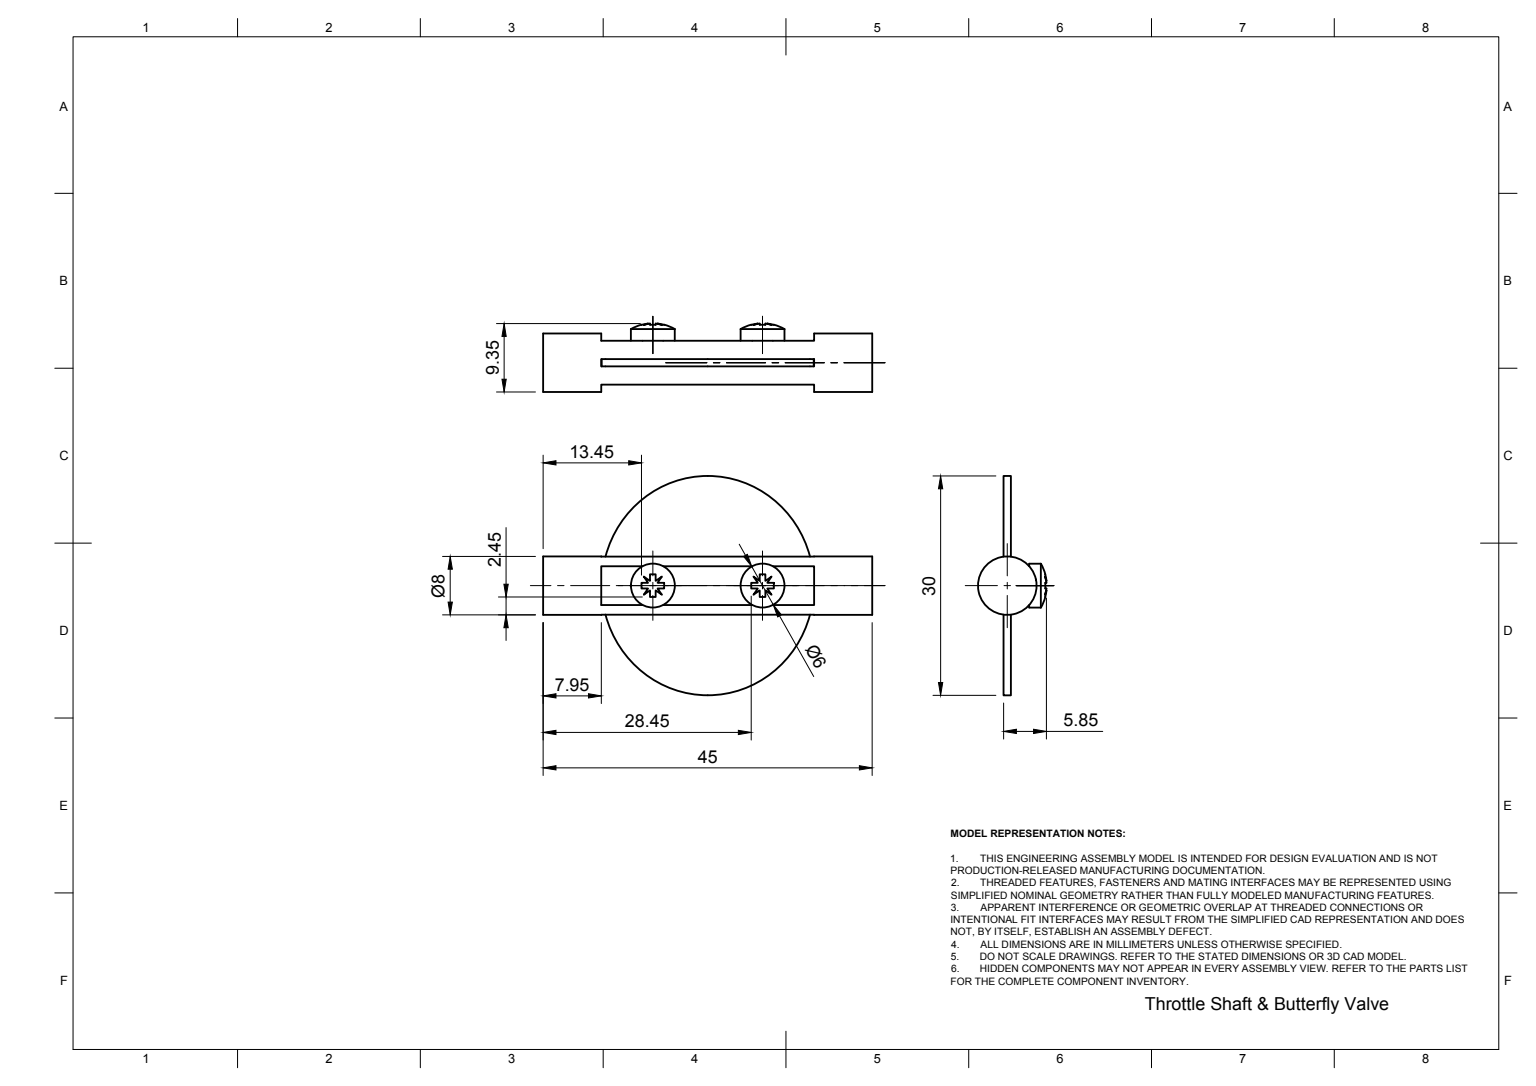
ISO-10303-21;
HEADER;
/* Generated by software containing ST-Developer
 * from STEP Tools, Inc. (www.steptools.com) 
 */

FILE_DESCRIPTION(
/* description */ ('STEP AP214'),
/* implementation_level */ '2;1');

FILE_NAME(
/* name */ 'Throttle Shaft & Butterfly Valve.step',
/* time_stamp */ '2026-10-07T12:18:07-07:00',
/* author */ (''),
/* organization */ (''),
/* preprocessor_version */ 'ST-DEVELOPER v20.2',
/* originating_system */ 'Autodesk Translation Framework v15.15.0.0',
/* authorisation */ '');

FILE_SCHEMA (('AUTOMOTIVE_DESIGN { 1 0 10303 214 3 1 1 }'));
ENDSEC;

DATA;
#10=MECHANICAL_DESIGN_GEOMETRIC_PRESENTATION_REPRESENTATION('',(#124),#62974);
#80=SPHERICAL_SURFACE('',#15545,6.);
#81=SPHERICAL_SURFACE('',#15579,6.);
#100=SHAPE_REPRESENTATION_RELATIONSHIP('SRR','None',#63023,#112);
#112=ADVANCED_BREP_SHAPE_REPRESENTATION('',(#136),#62964);
#124=STYLED_ITEM('',(#63090),#136);
#136=MANIFOLD_SOLID_BREP('Body1',#15194);
#147=(
BOUNDED_SURFACE()
B_SPLINE_SURFACE(3,1,((#34070,#34071),(#34072,#34073),(#34074,#34075),(#34076,
#34077)),.UNSPECIFIED.,.F.,.F.,.F.)
B_SPLINE_SURFACE_WITH_KNOTS((4,4),(2,2),(0.,1.),(0.,0.12),.UNSPECIFIED.)
GEOMETRIC_REPRESENTATION_ITEM()
RATIONAL_B_SPLINE_SURFACE(((1.,1.),(0.333333333333333,0.333333333333333),
(0.333333333333333,0.333333333333333),(1.,1.)))
REPRESENTATION_ITEM('')
SURFACE()
);
#148=(
BOUNDED_SURFACE()
B_SPLINE_SURFACE(3,1,((#34465,#34466),(#34467,#34468),(#34469,#34470),(#34471,
#34472)),.UNSPECIFIED.,.F.,.F.,.F.)
B_SPLINE_SURFACE_WITH_KNOTS((4,4),(2,2),(0.,1.),(0.,0.120000000000004),
 .UNSPECIFIED.)
GEOMETRIC_REPRESENTATION_ITEM()
RATIONAL_B_SPLINE_SURFACE(((1.,1.),(0.333333333333333,0.333333333333333),
(0.333333333333333,0.333333333333333),(1.,1.)))
REPRESENTATION_ITEM('')
SURFACE()
);
#212=FACE_BOUND('',#4694,.T.);
#213=FACE_BOUND('',#4696,.T.);
#214=FACE_BOUND('',#4697,.T.);
#215=FACE_BOUND('',#4698,.T.);
#216=FACE_BOUND('',#4700,.T.);
#365=PLANE('',#15607);
#366=PLANE('',#15609);
#367=PLANE('',#15610);
#368=PLANE('',#15612);
#369=PLANE('',#15613);
#370=PLANE('',#15614);
#371=PLANE('',#15615);
#372=PLANE('',#15616);
#373=PLANE('',#15617);
#374=PLANE('',#15618);
#375=PLANE('',#15619);
#376=PLANE('',#15620);
#377=PLANE('',#15621);
#378=PLANE('',#15622);
#379=PLANE('',#15623);
#380=PLANE('',#15624);
#381=PLANE('',#15625);
#382=PLANE('',#15626);
#383=PLANE('',#15627);
#384=PLANE('',#15628);
#385=PLANE('',#15629);
#386=PLANE('',#15630);
#387=PLANE('',#15631);
#388=PLANE('',#15632);
#389=PLANE('',#15633);
#390=PLANE('',#15634);
#391=PLANE('',#15635);
#392=PLANE('',#15636);
#393=PLANE('',#15637);
#394=PLANE('',#15638);
#395=PLANE('',#15639);
#396=PLANE('',#15640);
#397=PLANE('',#15641);
#398=PLANE('',#15642);
#399=PLANE('',#15643);
#400=PLANE('',#15644);
#401=PLANE('',#15645);
#402=PLANE('',#15646);
#403=PLANE('',#15647);
#404=PLANE('',#15648);
#405=PLANE('',#15649);
#406=PLANE('',#15650);
#407=PLANE('',#15651);
#408=PLANE('',#15652);
#409=PLANE('',#15653);
#410=PLANE('',#15654);
#411=PLANE('',#15655);
#412=PLANE('',#15656);
#413=PLANE('',#15657);
#414=PLANE('',#15658);
#415=PLANE('',#15659);
#416=PLANE('',#15660);
#417=PLANE('',#15661);
#418=PLANE('',#15662);
#419=PLANE('',#15663);
#420=PLANE('',#15664);
#421=PLANE('',#15665);
#422=PLANE('',#15666);
#423=PLANE('',#15667);
#424=PLANE('',#15668);
#425=PLANE('',#15669);
#426=PLANE('',#15670);
#427=PLANE('',#15671);
#428=PLANE('',#15673);
#429=PLANE('',#15675);
#430=PLANE('',#15678);
#739=ELLIPSE('',#15532,14.9999999999992,14.4999999999993);
#740=ELLIPSE('',#15533,15.0000000000004,14.5000000000004);
#741=ELLIPSE('',#15534,14.9999999999913,14.4999999999828);
#742=ELLIPSE('',#15535,15.0000000000001,14.5000000000001);
#743=ELLIPSE('',#15536,15.,14.5);
#744=ELLIPSE('',#15537,14.9999999999864,14.4999999999732);
#745=ELLIPSE('',#15608,14.9999999999937,14.4999999999875);
#746=ELLIPSE('',#15611,15.0000000000065,14.5000000000128);
#747=ELLIPSE('',#15672,15.0000000000007,14.5000000000006);
#748=ELLIPSE('',#15674,15.0000000000004,14.5000000000003);
#749=ELLIPSE('',#15676,15.0000000000002,14.5000000000001);
#750=ELLIPSE('',#15677,15.0000000000002,14.5000000000002);
#1237=LINE('',#34082,#2430);
#1238=LINE('',#34090,#2431);
#1239=LINE('',#34103,#2432);
#1240=LINE('',#34153,#2433);
#1241=LINE('',#34156,#2434);
#1242=LINE('',#34158,#2435);
#1243=LINE('',#34160,#2436);
#1244=LINE('',#34164,#2437);
#1245=LINE('',#34169,#2438);
#1246=LINE('',#34170,#2439);
#1247=LINE('',#34172,#2440);
#1248=LINE('',#34178,#2441);
#1249=LINE('',#34179,#2442);
#1250=LINE('',#34181,#2443);
#1251=LINE('',#34184,#2444);
#1252=LINE('',#34186,#2445);
#1253=LINE('',#34187,#2446);
#1254=LINE('',#34192,#2447);
#1255=LINE('',#34195,#2448);
#1256=LINE('',#34199,#2449);
#1257=LINE('',#34200,#2450);
#1258=LINE('',#34202,#2451);
#1259=LINE('',#34204,#2452);
#1260=LINE('',#34206,#2453);
#1261=LINE('',#34210,#2454);
#1262=LINE('',#34212,#2455);
#1263=LINE('',#34213,#2456);
#1264=LINE('',#34214,#2457);
#1265=LINE('',#34215,#2458);
#1266=LINE('',#34264,#2459);
#1267=LINE('',#34269,#2460);
#1268=LINE('',#34271,#2461);
#1269=LINE('',#34274,#2462);
#1270=LINE('',#34278,#2463);
#1271=LINE('',#34280,#2464);
#1272=LINE('',#34281,#2465);
#1273=LINE('',#34284,#2466);
#1274=LINE('',#34285,#2467);
#1275=LINE('',#34288,#2468);
#1276=LINE('',#34290,#2469);
#1277=LINE('',#34292,#2470);
#1278=LINE('',#34294,#2471);
#1279=LINE('',#34296,#2472);
#1280=LINE('',#34298,#2473);
#1281=LINE('',#34300,#2474);
#1282=LINE('',#34302,#2475);
#1283=LINE('',#34304,#2476);
#1284=LINE('',#34306,#2477);
#1285=LINE('',#34308,#2478);
#1286=LINE('',#34310,#2479);
#1287=LINE('',#34312,#2480);
#1288=LINE('',#34314,#2481);
#1289=LINE('',#34316,#2482);
#1290=LINE('',#34318,#2483);
#1291=LINE('',#34320,#2484);
#1292=LINE('',#34321,#2485);
#1293=LINE('',#34323,#2486);
#1294=LINE('',#34324,#2487);
#1295=LINE('',#34326,#2488);
#1296=LINE('',#34328,#2489);
#1297=LINE('',#34330,#2490);
#1298=LINE('',#34332,#2491);
#1299=LINE('',#34334,#2492);
#1300=LINE('',#34336,#2493);
#1301=LINE('',#34338,#2494);
#1302=LINE('',#34340,#2495);
#1303=LINE('',#34342,#2496);
#1304=LINE('',#34344,#2497);
#1305=LINE('',#34346,#2498);
#1306=LINE('',#34348,#2499);
#1307=LINE('',#34350,#2500);
#1308=LINE('',#34352,#2501);
#1309=LINE('',#34354,#2502);
#1310=LINE('',#34359,#2503);
#1311=LINE('',#34363,#2504);
#1312=LINE('',#34367,#2505);
#1313=LINE('',#34371,#2506);
#1314=LINE('',#34373,#2507);
#1315=LINE('',#34379,#2508);
#1316=LINE('',#34381,#2509);
#1317=LINE('',#34383,#2510);
#1318=LINE('',#34385,#2511);
#1319=LINE('',#34387,#2512);
#1320=LINE('',#34389,#2513);
#1321=LINE('',#34391,#2514);
#1322=LINE('',#34393,#2515);
#1323=LINE('',#34395,#2516);
#1324=LINE('',#34397,#2517);
#1325=LINE('',#34399,#2518);
#1326=LINE('',#34401,#2519);
#1327=LINE('',#34403,#2520);
#1328=LINE('',#34405,#2521);
#1329=LINE('',#34407,#2522);
#1330=LINE('',#34409,#2523);
#1331=LINE('',#34411,#2524);
#1332=LINE('',#34413,#2525);
#1333=LINE('',#34415,#2526);
#1334=LINE('',#34416,#2527);
#1335=LINE('',#34418,#2528);
#1336=LINE('',#34419,#2529);
#1337=LINE('',#34421,#2530);
#1338=LINE('',#34423,#2531);
#1339=LINE('',#34425,#2532);
#1340=LINE('',#34427,#2533);
#1341=LINE('',#34429,#2534);
#1342=LINE('',#34431,#2535);
#1343=LINE('',#34433,#2536);
#1344=LINE('',#34435,#2537);
#1345=LINE('',#34437,#2538);
#1346=LINE('',#34439,#2539);
#1347=LINE('',#34441,#2540);
#1348=LINE('',#34443,#2541);
#1349=LINE('',#34445,#2542);
#1350=LINE('',#34447,#2543);
#1351=LINE('',#34449,#2544);
#1352=LINE('',#34451,#2545);
#1353=LINE('',#34453,#2546);
#1354=LINE('',#34455,#2547);
#2430=VECTOR('',#17528,1000.);
#2431=VECTOR('',#17535,1000.);
#2432=VECTOR('',#17548,3.);
#2433=VECTOR('',#17601,4.);
#2434=VECTOR('',#17604,1000.);
#2435=VECTOR('',#17605,1000.);
#2436=VECTOR('',#17606,1000.);
#2437=VECTOR('',#17609,4.);
#2438=VECTOR('',#17614,1000.);
#2439=VECTOR('',#17615,1000.);
#2440=VECTOR('',#17616,1000.);
#2441=VECTOR('',#17621,1000.);
#2442=VECTOR('',#17622,1000.);
#2443=VECTOR('',#17623,1000.);
#2444=VECTOR('',#17626,1000.);
#2445=VECTOR('',#17627,1000.);
#2446=VECTOR('',#17628,1000.);
#2447=VECTOR('',#17631,1000.);
#2448=VECTOR('',#17634,1000.);
#2449=VECTOR('',#17637,1000.);
#2450=VECTOR('',#17638,1000.);
#2451=VECTOR('',#17639,1000.);
#2452=VECTOR('',#17640,1000.);
#2453=VECTOR('',#17641,1000.);
#2454=VECTOR('',#17644,1000.);
#2455=VECTOR('',#17645,1000.);
#2456=VECTOR('',#17646,1000.);
#2457=VECTOR('',#17647,1000.);
#2458=VECTOR('',#17648,1000.);
#2459=VECTOR('',#17701,3.);
#2460=VECTOR('',#17710,1000.);
#2461=VECTOR('',#17713,1000.);
#2462=VECTOR('',#17718,1000.);
#2463=VECTOR('',#17723,1000.);
#2464=VECTOR('',#17724,1000.);
#2465=VECTOR('',#17725,1000.);
#2466=VECTOR('',#17728,1000.);
#2467=VECTOR('',#17729,1000.);
#2468=VECTOR('',#17732,1000.);
#2469=VECTOR('',#17733,1000.);
#2470=VECTOR('',#17734,1000.);
#2471=VECTOR('',#17735,1000.);
#2472=VECTOR('',#17736,1000.);
#2473=VECTOR('',#17737,1000.);
#2474=VECTOR('',#17738,1000.);
#2475=VECTOR('',#17739,1000.);
#2476=VECTOR('',#17740,1000.);
#2477=VECTOR('',#17741,1000.);
#2478=VECTOR('',#17742,1000.);
#2479=VECTOR('',#17743,1000.);
#2480=VECTOR('',#17744,1000.);
#2481=VECTOR('',#17745,1000.);
#2482=VECTOR('',#17746,1000.);
#2483=VECTOR('',#17747,1000.);
#2484=VECTOR('',#17748,1000.);
#2485=VECTOR('',#17749,1000.);
#2486=VECTOR('',#17752,1000.);
#2487=VECTOR('',#17753,1000.);
#2488=VECTOR('',#17756,1000.);
#2489=VECTOR('',#17759,1000.);
#2490=VECTOR('',#17762,1000.);
#2491=VECTOR('',#17765,1000.);
#2492=VECTOR('',#17768,1000.);
#2493=VECTOR('',#17771,1000.);
#2494=VECTOR('',#17774,1000.);
#2495=VECTOR('',#17777,1000.);
#2496=VECTOR('',#17780,1000.);
#2497=VECTOR('',#17783,1000.);
#2498=VECTOR('',#17786,1000.);
#2499=VECTOR('',#17789,1000.);
#2500=VECTOR('',#17792,1000.);
#2501=VECTOR('',#17795,1000.);
#2502=VECTOR('',#17798,1000.);
#2503=VECTOR('',#17807,1000.);
#2504=VECTOR('',#17814,1000.);
#2505=VECTOR('',#17821,1000.);
#2506=VECTOR('',#17828,1000.);
#2507=VECTOR('',#17831,1000.);
#2508=VECTOR('',#17838,1000.);
#2509=VECTOR('',#17839,1000.);
#2510=VECTOR('',#17840,1000.);
#2511=VECTOR('',#17841,1000.);
#2512=VECTOR('',#17842,1000.);
#2513=VECTOR('',#17843,1000.);
#2514=VECTOR('',#17844,1000.);
#2515=VECTOR('',#17845,1000.);
#2516=VECTOR('',#17846,1000.);
#2517=VECTOR('',#17847,1000.);
#2518=VECTOR('',#17848,1000.);
#2519=VECTOR('',#17849,1000.);
#2520=VECTOR('',#17850,1000.);
#2521=VECTOR('',#17851,1000.);
#2522=VECTOR('',#17852,1000.);
#2523=VECTOR('',#17853,1000.);
#2524=VECTOR('',#17854,1000.);
#2525=VECTOR('',#17855,1000.);
#2526=VECTOR('',#17856,1000.);
#2527=VECTOR('',#17857,1000.);
#2528=VECTOR('',#17860,1000.);
#2529=VECTOR('',#17861,1000.);
#2530=VECTOR('',#17864,1000.);
#2531=VECTOR('',#17867,1000.);
#2532=VECTOR('',#17870,1000.);
#2533=VECTOR('',#17873,1000.);
#2534=VECTOR('',#17876,1000.);
#2535=VECTOR('',#17879,1000.);
#2536=VECTOR('',#17882,1000.);
#2537=VECTOR('',#17885,1000.);
#2538=VECTOR('',#17888,1000.);
#2539=VECTOR('',#17891,1000.);
#2540=VECTOR('',#17894,1000.);
#2541=VECTOR('',#17897,1000.);
#2542=VECTOR('',#17900,1000.);
#2543=VECTOR('',#17903,1000.);
#2544=VECTOR('',#17906,1000.);
#2545=VECTOR('',#17909,1000.);
#2546=VECTOR('',#17912,1000.);
#2547=VECTOR('',#17915,1000.);
#3461=CYLINDRICAL_SURFACE('',#15538,3.);
#3462=CYLINDRICAL_SURFACE('',#15566,4.);
#3463=CYLINDRICAL_SURFACE('',#15601,3.);
#3806=FACE_OUTER_BOUND('',#4691,.T.);
#3807=FACE_OUTER_BOUND('',#4692,.T.);
#3808=FACE_OUTER_BOUND('',#4693,.T.);
#3809=FACE_OUTER_BOUND('',#4695,.T.);
#3810=FACE_OUTER_BOUND('',#4699,.T.);
#3811=FACE_OUTER_BOUND('',#4701,.T.);
#3812=FACE_OUTER_BOUND('',#4702,.T.);
#3813=FACE_OUTER_BOUND('',#4703,.T.);
#3814=FACE_OUTER_BOUND('',#4704,.T.);
#3815=FACE_OUTER_BOUND('',#4705,.T.);
#3816=FACE_OUTER_BOUND('',#4706,.T.);
#3817=FACE_OUTER_BOUND('',#4707,.T.);
#3818=FACE_OUTER_BOUND('',#4708,.T.);
#3819=FACE_OUTER_BOUND('',#4709,.T.);
#3820=FACE_OUTER_BOUND('',#4710,.T.);
#3821=FACE_OUTER_BOUND('',#4711,.T.);
#3822=FACE_OUTER_BOUND('',#4712,.T.);
#3823=FACE_OUTER_BOUND('',#4713,.T.);
#3824=FACE_OUTER_BOUND('',#4714,.T.);
#3825=FACE_OUTER_BOUND('',#4715,.T.);
#3826=FACE_OUTER_BOUND('',#4716,.T.);
#3827=FACE_OUTER_BOUND('',#4717,.T.);
#3828=FACE_OUTER_BOUND('',#4718,.T.);
#3829=FACE_OUTER_BOUND('',#4719,.T.);
#3830=FACE_OUTER_BOUND('',#4720,.T.);
#3831=FACE_OUTER_BOUND('',#4721,.T.);
#3832=FACE_OUTER_BOUND('',#4722,.T.);
#3833=FACE_OUTER_BOUND('',#4723,.T.);
#3834=FACE_OUTER_BOUND('',#4724,.T.);
#3835=FACE_OUTER_BOUND('',#4725,.T.);
#3836=FACE_OUTER_BOUND('',#4726,.T.);
#3837=FACE_OUTER_BOUND('',#4727,.T.);
#3838=FACE_OUTER_BOUND('',#4728,.T.);
#3839=FACE_OUTER_BOUND('',#4729,.T.);
#3840=FACE_OUTER_BOUND('',#4730,.T.);
#3841=FACE_OUTER_BOUND('',#4731,.T.);
#3842=FACE_OUTER_BOUND('',#4732,.T.);
#3843=FACE_OUTER_BOUND('',#4733,.T.);
#3844=FACE_OUTER_BOUND('',#4734,.T.);
#3845=FACE_OUTER_BOUND('',#4735,.T.);
#3846=FACE_OUTER_BOUND('',#4736,.T.);
#3847=FACE_OUTER_BOUND('',#4737,.T.);
#3848=FACE_OUTER_BOUND('',#4738,.T.);
#3849=FACE_OUTER_BOUND('',#4739,.T.);
#3850=FACE_OUTER_BOUND('',#4740,.T.);
#3851=FACE_OUTER_BOUND('',#4741,.T.);
#3852=FACE_OUTER_BOUND('',#4742,.T.);
#3853=FACE_OUTER_BOUND('',#4743,.T.);
#3854=FACE_OUTER_BOUND('',#4744,.T.);
#3855=FACE_OUTER_BOUND('',#4745,.T.);
#3856=FACE_OUTER_BOUND('',#4746,.T.);
#3857=FACE_OUTER_BOUND('',#4747,.T.);
#3858=FACE_OUTER_BOUND('',#4748,.T.);
#3859=FACE_OUTER_BOUND('',#4749,.T.);
#3860=FACE_OUTER_BOUND('',#4750,.T.);
#3861=FACE_OUTER_BOUND('',#4751,.T.);
#3862=FACE_OUTER_BOUND('',#4752,.T.);
#3863=FACE_OUTER_BOUND('',#4753,.T.);
#3864=FACE_OUTER_BOUND('',#4754,.T.);
#3865=FACE_OUTER_BOUND('',#4755,.T.);
#3866=FACE_OUTER_BOUND('',#4756,.T.);
#3867=FACE_OUTER_BOUND('',#4757,.T.);
#3868=FACE_OUTER_BOUND('',#4758,.T.);
#3869=FACE_OUTER_BOUND('',#4759,.T.);
#3870=FACE_OUTER_BOUND('',#4760,.T.);
#3871=FACE_OUTER_BOUND('',#4761,.T.);
#3872=FACE_OUTER_BOUND('',#4762,.T.);
#3873=FACE_OUTER_BOUND('',#4763,.T.);
#3874=FACE_OUTER_BOUND('',#4764,.T.);
#3875=FACE_OUTER_BOUND('',#4765,.T.);
#3876=FACE_OUTER_BOUND('',#4766,.T.);
#3877=FACE_OUTER_BOUND('',#4767,.T.);
#3878=FACE_OUTER_BOUND('',#4768,.T.);
#4691=EDGE_LOOP('',(#10355,#10356,#10357,#10358,#10359,#10360,#10361,#10362));
#4692=EDGE_LOOP('',(#10363,#10364,#10365,#10366,#10367,#10368,#10369,#10370));
#4693=EDGE_LOOP('',(#10371));
#4694=EDGE_LOOP('',(#10372,#10373,#10374,#10375,#10376,#10377,#10378,#10379,
#10380,#10381,#10382,#10383,#10384,#10385,#10386,#10387,#10388,#10389,#10390,
#10391));
#4695=EDGE_LOOP('',(#10392,#10393,#10394,#10395,#10396,#10397,#10398,#10399,
#10400,#10401,#10402,#10403,#10404,#10405,#10406,#10407));
#4696=EDGE_LOOP('',(#10408,#10409,#10410,#10411,#10412,#10413,#10414,#10415));
#4697=EDGE_LOOP('',(#10416,#10417,#10418,#10419));
#4698=EDGE_LOOP('',(#10420,#10421,#10422,#10423,#10424,#10425,#10426,#10427,
#10428,#10429,#10430,#10431));
#4699=EDGE_LOOP('',(#10432));
#4700=EDGE_LOOP('',(#10433,#10434,#10435,#10436,#10437,#10438,#10439,#10440,
#10441,#10442,#10443,#10444,#10445,#10446,#10447,#10448,#10449,#10450,#10451,
#10452));
#4701=EDGE_LOOP('',(#10453,#10454,#10455,#10456,#10457,#10458,#10459,#10460));
#4702=EDGE_LOOP('',(#10461,#10462,#10463,#10464));
#4703=EDGE_LOOP('',(#10465,#10466,#10467,#10468));
#4704=EDGE_LOOP('',(#10469,#10470,#10471,#10472));
#4705=EDGE_LOOP('',(#10473,#10474,#10475));
#4706=EDGE_LOOP('',(#10476,#10477,#10478,#10479));
#4707=EDGE_LOOP('',(#10480,#10481,#10482,#10483));
#4708=EDGE_LOOP('',(#10484,#10485,#10486,#10487,#10488,#10489,#10490,#10491,
#10492,#10493,#10494,#10495,#10496,#10497,#10498,#10499,#10500,#10501,#10502,
#10503));
#4709=EDGE_LOOP('',(#10504,#10505,#10506,#10507));
#4710=EDGE_LOOP('',(#10508,#10509,#10510,#10511));
#4711=EDGE_LOOP('',(#10512,#10513,#10514,#10515));
#4712=EDGE_LOOP('',(#10516,#10517,#10518,#10519));
#4713=EDGE_LOOP('',(#10520,#10521,#10522,#10523));
#4714=EDGE_LOOP('',(#10524,#10525,#10526,#10527));
#4715=EDGE_LOOP('',(#10528,#10529,#10530,#10531));
#4716=EDGE_LOOP('',(#10532,#10533,#10534,#10535));
#4717=EDGE_LOOP('',(#10536,#10537,#10538,#10539));
#4718=EDGE_LOOP('',(#10540,#10541,#10542,#10543));
#4719=EDGE_LOOP('',(#10544,#10545,#10546,#10547));
#4720=EDGE_LOOP('',(#10548,#10549,#10550,#10551));
#4721=EDGE_LOOP('',(#10552,#10553,#10554,#10555));
#4722=EDGE_LOOP('',(#10556,#10557,#10558,#10559));
#4723=EDGE_LOOP('',(#10560,#10561,#10562,#10563));
#4724=EDGE_LOOP('',(#10564,#10565,#10566,#10567));
#4725=EDGE_LOOP('',(#10568,#10569,#10570,#10571));
#4726=EDGE_LOOP('',(#10572,#10573,#10574,#10575));
#4727=EDGE_LOOP('',(#10576,#10577));
#4728=EDGE_LOOP('',(#10578,#10579,#10580,#10581));
#4729=EDGE_LOOP('',(#10582,#10583,#10584,#10585));
#4730=EDGE_LOOP('',(#10586));
#4731=EDGE_LOOP('',(#10587,#10588,#10589,#10590,#10591));
#4732=EDGE_LOOP('',(#10592,#10593));
#4733=EDGE_LOOP('',(#10594));
#4734=EDGE_LOOP('',(#10595,#10596,#10597,#10598));
#4735=EDGE_LOOP('',(#10599,#10600));
#4736=EDGE_LOOP('',(#10601,#10602,#10603,#10604,#10605));
#4737=EDGE_LOOP('',(#10606,#10607));
#4738=EDGE_LOOP('',(#10608,#10609,#10610,#10611));
#4739=EDGE_LOOP('',(#10612,#10613));
#4740=EDGE_LOOP('',(#10614,#10615,#10616,#10617));
#4741=EDGE_LOOP('',(#10618,#10619,#10620,#10621,#10622,#10623,#10624,#10625,
#10626,#10627,#10628,#10629,#10630,#10631,#10632,#10633,#10634,#10635,#10636,
#10637));
#4742=EDGE_LOOP('',(#10638,#10639,#10640,#10641));
#4743=EDGE_LOOP('',(#10642,#10643,#10644,#10645));
#4744=EDGE_LOOP('',(#10646,#10647,#10648,#10649));
#4745=EDGE_LOOP('',(#10650,#10651,#10652,#10653));
#4746=EDGE_LOOP('',(#10654,#10655,#10656,#10657));
#4747=EDGE_LOOP('',(#10658,#10659,#10660,#10661));
#4748=EDGE_LOOP('',(#10662,#10663,#10664,#10665));
#4749=EDGE_LOOP('',(#10666,#10667,#10668,#10669));
#4750=EDGE_LOOP('',(#10670,#10671,#10672,#10673));
#4751=EDGE_LOOP('',(#10674,#10675,#10676,#10677));
#4752=EDGE_LOOP('',(#10678,#10679,#10680,#10681));
#4753=EDGE_LOOP('',(#10682,#10683,#10684,#10685));
#4754=EDGE_LOOP('',(#10686,#10687,#10688,#10689));
#4755=EDGE_LOOP('',(#10690,#10691,#10692,#10693));
#4756=EDGE_LOOP('',(#10694,#10695,#10696,#10697));
#4757=EDGE_LOOP('',(#10698,#10699,#10700,#10701));
#4758=EDGE_LOOP('',(#10702,#10703,#10704,#10705));
#4759=EDGE_LOOP('',(#10706,#10707,#10708,#10709));
#4760=EDGE_LOOP('',(#10710,#10711,#10712,#10713));
#4761=EDGE_LOOP('',(#10714,#10715,#10716,#10717));
#4762=EDGE_LOOP('',(#10718,#10719));
#4763=EDGE_LOOP('',(#10720,#10721,#10722));
#4764=EDGE_LOOP('',(#10723,#10724,#10725));
#4765=EDGE_LOOP('',(#10726,#10727,#10728));
#4766=EDGE_LOOP('',(#10729,#10730,#10731));
#4767=EDGE_LOOP('',(#10732,#10733,#10734,#10735,#10736,#10737,#10738,#10739));
#4768=EDGE_LOOP('',(#10740,#10741,#10742));
#5583=CIRCLE('',#15539,3.);
#5584=CIRCLE('',#15540,3.);
#5585=CIRCLE('',#15541,3.);
#5586=CIRCLE('',#15542,3.);
#5587=CIRCLE('',#15543,3.);
#5588=CIRCLE('',#15544,3.);
#5589=CIRCLE('',#15546,5.7963350489771);
#5590=CIRCLE('',#15547,5.98747390390977);
#5591=CIRCLE('',#15548,5.99149706962117);
#5592=CIRCLE('',#15549,5.99149706962117);
#5593=CIRCLE('',#15550,5.98747390390977);
#5594=CIRCLE('',#15551,5.79633504897711);
#5595=CIRCLE('',#15552,5.98747390390978);
#5596=CIRCLE('',#15553,5.99149706962117);
#5597=CIRCLE('',#15554,5.99149706962117);
#5598=CIRCLE('',#15555,5.98747390390977);
#5599=CIRCLE('',#15556,5.79633504897713);
#5600=CIRCLE('',#15557,5.98747390390977);
#5601=CIRCLE('',#15558,5.99149706962117);
#5602=CIRCLE('',#15559,5.99149706962117);
#5603=CIRCLE('',#15560,5.98747390390978);
#5604=CIRCLE('',#15561,5.79633504897711);
#5605=CIRCLE('',#15562,5.98747390390977);
#5606=CIRCLE('',#15563,5.99149706962117);
#5607=CIRCLE('',#15564,5.99149706962117);
#5608=CIRCLE('',#15565,5.98747390390977);
#5609=CIRCLE('',#15567,4.);
#5610=CIRCLE('',#15568,4.);
#5611=CIRCLE('',#15569,4.);
#5612=CIRCLE('',#15570,4.);
#5613=CIRCLE('',#15571,4.);
#5614=CIRCLE('',#15572,4.);
#5615=CIRCLE('',#15573,4.);
#5616=CIRCLE('',#15574,4.);
#5617=CIRCLE('',#15575,4.);
#5618=CIRCLE('',#15576,4.);
#5619=CIRCLE('',#15577,4.);
#5620=CIRCLE('',#15578,4.);
#5621=CIRCLE('',#15580,3.);
#5622=CIRCLE('',#15581,5.7963350489771);
#5623=CIRCLE('',#15582,5.98747390390977);
#5624=CIRCLE('',#15583,5.99149706962117);
#5625=CIRCLE('',#15584,5.99149706962117);
#5626=CIRCLE('',#15585,5.98747390390977);
#5627=CIRCLE('',#15586,5.79633504897711);
#5628=CIRCLE('',#15587,5.98747390390978);
#5629=CIRCLE('',#15588,5.99149706962117);
#5630=CIRCLE('',#15589,5.99149706962117);
#5631=CIRCLE('',#15590,5.98747390390977);
#5632=CIRCLE('',#15591,5.79633504897713);
#5633=CIRCLE('',#15592,5.98747390390977);
#5634=CIRCLE('',#15593,5.99149706962117);
#5635=CIRCLE('',#15594,5.99149706962117);
#5636=CIRCLE('',#15595,5.98747390390978);
#5637=CIRCLE('',#15596,5.79633504897711);
#5638=CIRCLE('',#15597,5.98747390390977);
#5639=CIRCLE('',#15598,5.99149706962117);
#5640=CIRCLE('',#15599,5.99149706962117);
#5641=CIRCLE('',#15600,5.98747390390977);
#5642=CIRCLE('',#15602,3.);
#5643=CIRCLE('',#15603,3.);
#5644=CIRCLE('',#15604,3.);
#5645=CIRCLE('',#15605,3.);
#5646=CIRCLE('',#15606,3.);
#6386=VERTEX_POINT('',#34078);
#6387=VERTEX_POINT('',#34079);
#6388=VERTEX_POINT('',#34081);
#6389=VERTEX_POINT('',#34083);
#6390=VERTEX_POINT('',#34085);
#6391=VERTEX_POINT('',#34087);
#6392=VERTEX_POINT('',#34089);
#6393=VERTEX_POINT('',#34091);
#6394=VERTEX_POINT('',#34095);
#6395=VERTEX_POINT('',#34096);
#6396=VERTEX_POINT('',#34098);
#6397=VERTEX_POINT('',#34100);
#6398=VERTEX_POINT('',#34102);
#6399=VERTEX_POINT('',#34105);
#6400=VERTEX_POINT('',#34109);
#6401=VERTEX_POINT('',#34110);
#6402=VERTEX_POINT('',#34112);
#6403=VERTEX_POINT('',#34114);
#6404=VERTEX_POINT('',#34116);
#6405=VERTEX_POINT('',#34118);
#6406=VERTEX_POINT('',#34120);
#6407=VERTEX_POINT('',#34122);
#6408=VERTEX_POINT('',#34124);
#6409=VERTEX_POINT('',#34126);
#6410=VERTEX_POINT('',#34128);
#6411=VERTEX_POINT('',#34130);
#6412=VERTEX_POINT('',#34132);
#6413=VERTEX_POINT('',#34134);
#6414=VERTEX_POINT('',#34136);
#6415=VERTEX_POINT('',#34138);
#6416=VERTEX_POINT('',#34140);
#6417=VERTEX_POINT('',#34142);
#6418=VERTEX_POINT('',#34144);
#6419=VERTEX_POINT('',#34146);
#6420=VERTEX_POINT('',#34150);
#6421=VERTEX_POINT('',#34152);
#6422=VERTEX_POINT('',#34154);
#6423=VERTEX_POINT('',#34157);
#6424=VERTEX_POINT('',#34159);
#6425=VERTEX_POINT('',#34161);
#6426=VERTEX_POINT('',#34163);
#6427=VERTEX_POINT('',#34166);
#6428=VERTEX_POINT('',#34168);
#6429=VERTEX_POINT('',#34171);
#6430=VERTEX_POINT('',#34174);
#6431=VERTEX_POINT('',#34175);
#6432=VERTEX_POINT('',#34177);
#6433=VERTEX_POINT('',#34180);
#6434=VERTEX_POINT('',#34182);
#6435=VERTEX_POINT('',#34185);
#6436=VERTEX_POINT('',#34188);
#6437=VERTEX_POINT('',#34189);
#6438=VERTEX_POINT('',#34191);
#6439=VERTEX_POINT('',#34193);
#6440=VERTEX_POINT('',#34196);
#6441=VERTEX_POINT('',#34197);
#6442=VERTEX_POINT('',#34201);
#6443=VERTEX_POINT('',#34203);
#6444=VERTEX_POINT('',#34205);
#6445=VERTEX_POINT('',#34207);
#6446=VERTEX_POINT('',#34209);
#6447=VERTEX_POINT('',#34211);
#6448=VERTEX_POINT('',#34217);
#6449=VERTEX_POINT('',#34219);
#6450=VERTEX_POINT('',#34220);
#6451=VERTEX_POINT('',#34222);
#6452=VERTEX_POINT('',#34224);
#6453=VERTEX_POINT('',#34226);
#6454=VERTEX_POINT('',#34228);
#6455=VERTEX_POINT('',#34230);
#6456=VERTEX_POINT('',#34232);
#6457=VERTEX_POINT('',#34234);
#6458=VERTEX_POINT('',#34236);
#6459=VERTEX_POINT('',#34238);
#6460=VERTEX_POINT('',#34240);
#6461=VERTEX_POINT('',#34242);
#6462=VERTEX_POINT('',#34244);
#6463=VERTEX_POINT('',#34246);
#6464=VERTEX_POINT('',#34248);
#6465=VERTEX_POINT('',#34250);
#6466=VERTEX_POINT('',#34252);
#6467=VERTEX_POINT('',#34254);
#6468=VERTEX_POINT('',#34256);
#6469=VERTEX_POINT('',#34262);
#6470=VERTEX_POINT('',#34277);
#6471=VERTEX_POINT('',#34279);
#6472=VERTEX_POINT('',#34283);
#6473=VERTEX_POINT('',#34287);
#6474=VERTEX_POINT('',#34289);
#6475=VERTEX_POINT('',#34291);
#6476=VERTEX_POINT('',#34293);
#6477=VERTEX_POINT('',#34295);
#6478=VERTEX_POINT('',#34297);
#6479=VERTEX_POINT('',#34299);
#6480=VERTEX_POINT('',#34301);
#6481=VERTEX_POINT('',#34303);
#6482=VERTEX_POINT('',#34305);
#6483=VERTEX_POINT('',#34307);
#6484=VERTEX_POINT('',#34309);
#6485=VERTEX_POINT('',#34311);
#6486=VERTEX_POINT('',#34313);
#6487=VERTEX_POINT('',#34315);
#6488=VERTEX_POINT('',#34317);
#6489=VERTEX_POINT('',#34319);
#6490=VERTEX_POINT('',#34377);
#6491=VERTEX_POINT('',#34378);
#6492=VERTEX_POINT('',#34380);
#6493=VERTEX_POINT('',#34382);
#6494=VERTEX_POINT('',#34384);
#6495=VERTEX_POINT('',#34386);
#6496=VERTEX_POINT('',#34388);
#6497=VERTEX_POINT('',#34390);
#6498=VERTEX_POINT('',#34392);
#6499=VERTEX_POINT('',#34394);
#6500=VERTEX_POINT('',#34396);
#6501=VERTEX_POINT('',#34398);
#6502=VERTEX_POINT('',#34400);
#6503=VERTEX_POINT('',#34402);
#6504=VERTEX_POINT('',#34404);
#6505=VERTEX_POINT('',#34406);
#6506=VERTEX_POINT('',#34408);
#6507=VERTEX_POINT('',#34410);
#6508=VERTEX_POINT('',#34412);
#6509=VERTEX_POINT('',#34414);
#7884=EDGE_CURVE('',#6386,#6387,#739,.T.);
#7885=EDGE_CURVE('',#6386,#6388,#1237,.T.);
#7886=EDGE_CURVE('',#6388,#6389,#740,.T.);
#7887=EDGE_CURVE('',#6389,#6390,#741,.T.);
#7888=EDGE_CURVE('',#6390,#6391,#742,.T.);
#7889=EDGE_CURVE('',#6392,#6391,#1238,.T.);
#7890=EDGE_CURVE('',#6393,#6392,#743,.T.);
#7891=EDGE_CURVE('',#6387,#6393,#744,.T.);
#7892=EDGE_CURVE('',#6394,#6395,#5583,.T.);
#7893=EDGE_CURVE('',#6395,#6396,#5584,.T.);
#7894=EDGE_CURVE('',#6396,#6397,#5585,.T.);
#7895=EDGE_CURVE('',#6397,#6398,#1239,.T.);
#7896=EDGE_CURVE('',#6398,#6398,#5586,.T.);
#7897=EDGE_CURVE('',#6397,#6399,#5587,.T.);
#7898=EDGE_CURVE('',#6399,#6394,#5588,.T.);
#7899=EDGE_CURVE('',#6400,#6401,#5589,.T.);
#7900=EDGE_CURVE('',#6401,#6402,#5590,.T.);
#7901=EDGE_CURVE('',#6402,#6403,#5591,.T.);
#7902=EDGE_CURVE('',#6403,#6404,#5592,.T.);
#7903=EDGE_CURVE('',#6404,#6405,#5593,.T.);
#7904=EDGE_CURVE('',#6405,#6406,#5594,.T.);
#7905=EDGE_CURVE('',#6406,#6407,#5595,.T.);
#7906=EDGE_CURVE('',#6407,#6408,#5596,.T.);
#7907=EDGE_CURVE('',#6408,#6409,#5597,.T.);
#7908=EDGE_CURVE('',#6409,#6410,#5598,.T.);
#7909=EDGE_CURVE('',#6410,#6411,#5599,.T.);
#7910=EDGE_CURVE('',#6411,#6412,#5600,.T.);
#7911=EDGE_CURVE('',#6412,#6413,#5601,.T.);
#7912=EDGE_CURVE('',#6413,#6414,#5602,.T.);
#7913=EDGE_CURVE('',#6414,#6415,#5603,.T.);
#7914=EDGE_CURVE('',#6415,#6416,#5604,.T.);
#7915=EDGE_CURVE('',#6416,#6417,#5605,.T.);
#7916=EDGE_CURVE('',#6417,#6418,#5606,.T.);
#7917=EDGE_CURVE('',#6418,#6419,#5607,.T.);
#7918=EDGE_CURVE('',#6419,#6400,#5608,.T.);
#7919=EDGE_CURVE('',#6420,#6420,#5609,.T.);
#7920=EDGE_CURVE('',#6420,#6421,#1240,.T.);
#7921=EDGE_CURVE('',#6422,#6421,#5610,.T.);
#7922=EDGE_CURVE('',#6422,#6393,#1241,.T.);
#7923=EDGE_CURVE('',#6393,#6423,#1242,.T.);
#7924=EDGE_CURVE('',#6423,#6424,#1243,.T.);
#7925=EDGE_CURVE('',#6424,#6425,#5611,.T.);
#7926=EDGE_CURVE('',#6425,#6426,#1244,.T.);
#7927=EDGE_CURVE('',#6426,#6426,#5612,.T.);
#7928=EDGE_CURVE('',#6425,#6427,#5613,.T.);
#7929=EDGE_CURVE('',#6428,#6427,#1245,.T.);
#7930=EDGE_CURVE('',#6390,#6428,#1246,.T.);
#7931=EDGE_CURVE('',#6429,#6390,#1247,.T.);
#7932=EDGE_CURVE('',#6421,#6429,#5614,.T.);
#7933=EDGE_CURVE('',#6430,#6431,#5615,.T.);
#7934=EDGE_CURVE('',#6432,#6431,#1248,.T.);
#7935=EDGE_CURVE('',#6387,#6432,#1249,.T.);
#7936=EDGE_CURVE('',#6433,#6387,#1250,.T.);
#7937=EDGE_CURVE('',#6434,#6433,#5616,.T.);
#7938=EDGE_CURVE('',#6434,#6389,#1251,.T.);
#7939=EDGE_CURVE('',#6389,#6435,#1252,.T.);
#7940=EDGE_CURVE('',#6435,#6430,#1253,.T.);
#7941=EDGE_CURVE('',#6436,#6437,#5617,.T.);
#7942=EDGE_CURVE('',#6436,#6438,#1254,.T.);
#7943=EDGE_CURVE('',#6438,#6439,#5618,.T.);
#7944=EDGE_CURVE('',#6437,#6439,#1255,.T.);
#7945=EDGE_CURVE('',#6440,#6441,#5619,.T.);
#7946=EDGE_CURVE('',#6440,#6399,#1256,.T.);
#7947=EDGE_CURVE('',#6399,#6396,#1257,.T.);
#7948=EDGE_CURVE('',#6396,#6442,#1258,.T.);
#7949=EDGE_CURVE('',#6442,#6443,#1259,.T.);
#7950=EDGE_CURVE('',#6443,#6444,#1260,.T.);
#7951=EDGE_CURVE('',#6444,#6445,#5620,.T.);
#7952=EDGE_CURVE('',#6446,#6445,#1261,.T.);
#7953=EDGE_CURVE('',#6447,#6446,#1262,.T.);
#7954=EDGE_CURVE('',#6395,#6447,#1263,.T.);
#7955=EDGE_CURVE('',#6394,#6395,#1264,.T.);
#7956=EDGE_CURVE('',#6441,#6394,#1265,.T.);
#7957=EDGE_CURVE('',#6448,#6448,#5621,.T.);
#7958=EDGE_CURVE('',#6449,#6450,#5622,.T.);
#7959=EDGE_CURVE('',#6450,#6451,#5623,.T.);
#7960=EDGE_CURVE('',#6451,#6452,#5624,.T.);
#7961=EDGE_CURVE('',#6452,#6453,#5625,.T.);
#7962=EDGE_CURVE('',#6453,#6454,#5626,.T.);
#7963=EDGE_CURVE('',#6454,#6455,#5627,.T.);
#7964=EDGE_CURVE('',#6455,#6456,#5628,.T.);
#7965=EDGE_CURVE('',#6456,#6457,#5629,.T.);
#7966=EDGE_CURVE('',#6457,#6458,#5630,.T.);
#7967=EDGE_CURVE('',#6458,#6459,#5631,.T.);
#7968=EDGE_CURVE('',#6459,#6460,#5632,.T.);
#7969=EDGE_CURVE('',#6460,#6461,#5633,.T.);
#7970=EDGE_CURVE('',#6461,#6462,#5634,.T.);
#7971=EDGE_CURVE('',#6462,#6463,#5635,.T.);
#7972=EDGE_CURVE('',#6463,#6464,#5636,.T.);
#7973=EDGE_CURVE('',#6464,#6465,#5637,.T.);
#7974=EDGE_CURVE('',#6465,#6466,#5638,.T.);
#7975=EDGE_CURVE('',#6466,#6467,#5639,.T.);
#7976=EDGE_CURVE('',#6467,#6468,#5640,.T.);
#7977=EDGE_CURVE('',#6468,#6449,#5641,.T.);
#7978=EDGE_CURVE('',#6447,#6446,#5642,.T.);
#7979=EDGE_CURVE('',#6446,#6443,#5643,.T.);
#7980=EDGE_CURVE('',#6443,#6469,#5644,.T.);
#7981=EDGE_CURVE('',#6469,#6448,#1266,.T.);
#7982=EDGE_CURVE('',#6469,#6442,#5645,.T.);
#7983=EDGE_CURVE('',#6442,#6447,#5646,.T.);
#7984=EDGE_CURVE('',#6428,#6435,#745,.T.);
#7985=EDGE_CURVE('',#6427,#6430,#1267,.T.);
#7986=EDGE_CURVE('',#6429,#6434,#1268,.T.);
#7987=EDGE_CURVE('',#6423,#6432,#746,.T.);
#7988=EDGE_CURVE('',#6431,#6424,#1269,.T.);
#7989=EDGE_CURVE('',#6470,#6451,#1270,.T.);
#7990=EDGE_CURVE('',#6470,#6471,#1271,.T.);
#7991=EDGE_CURVE('',#6452,#6471,#1272,.T.);
#7992=EDGE_CURVE('',#6471,#6472,#1273,.T.);
#7993=EDGE_CURVE('',#6453,#6472,#1274,.T.);
#7994=EDGE_CURVE('',#6473,#6470,#1275,.T.);
#7995=EDGE_CURVE('',#6474,#6473,#1276,.T.);
#7996=EDGE_CURVE('',#6475,#6474,#1277,.T.);
#7997=EDGE_CURVE('',#6476,#6475,#1278,.T.);
#7998=EDGE_CURVE('',#6477,#6476,#1279,.T.);
#7999=EDGE_CURVE('',#6478,#6477,#1280,.T.);
#8000=EDGE_CURVE('',#6479,#6478,#1281,.T.);
#8001=EDGE_CURVE('',#6480,#6479,#1282,.T.);
#8002=EDGE_CURVE('',#6481,#6480,#1283,.T.);
#8003=EDGE_CURVE('',#6482,#6481,#1284,.T.);
#8004=EDGE_CURVE('',#6483,#6482,#1285,.T.);
#8005=EDGE_CURVE('',#6484,#6483,#1286,.T.);
#8006=EDGE_CURVE('',#6485,#6484,#1287,.T.);
#8007=EDGE_CURVE('',#6486,#6485,#1288,.T.);
#8008=EDGE_CURVE('',#6487,#6486,#1289,.T.);
#8009=EDGE_CURVE('',#6488,#6487,#1290,.T.);
#8010=EDGE_CURVE('',#6489,#6488,#1291,.T.);
#8011=EDGE_CURVE('',#6472,#6489,#1292,.T.);
#8012=EDGE_CURVE('',#6454,#6489,#1293,.T.);
#8013=EDGE_CURVE('',#6455,#6488,#1294,.T.);
#8014=EDGE_CURVE('',#6487,#6456,#1295,.T.);
#8015=EDGE_CURVE('',#6457,#6486,#1296,.T.);
#8016=EDGE_CURVE('',#6458,#6485,#1297,.T.);
#8017=EDGE_CURVE('',#6459,#6484,#1298,.T.);
#8018=EDGE_CURVE('',#6460,#6483,#1299,.T.);
#8019=EDGE_CURVE('',#6482,#6461,#1300,.T.);
#8020=EDGE_CURVE('',#6462,#6481,#1301,.T.);
#8021=EDGE_CURVE('',#6463,#6480,#1302,.T.);
#8022=EDGE_CURVE('',#6464,#6479,#1303,.T.);
#8023=EDGE_CURVE('',#6465,#6478,#1304,.T.);
#8024=EDGE_CURVE('',#6477,#6466,#1305,.T.);
#8025=EDGE_CURVE('',#6467,#6476,#1306,.T.);
#8026=EDGE_CURVE('',#6468,#6475,#1307,.T.);
#8027=EDGE_CURVE('',#6449,#6474,#1308,.T.);
#8028=EDGE_CURVE('',#6450,#6473,#1309,.T.);
#8029=EDGE_CURVE('',#6445,#6444,#1310,.T.);
#8030=EDGE_CURVE('',#6433,#6422,#1311,.T.);
#8031=EDGE_CURVE('',#6441,#6440,#1312,.T.);
#8032=EDGE_CURVE('',#6439,#6438,#1313,.T.);
#8033=EDGE_CURVE('',#6437,#6436,#1314,.T.);
#8034=EDGE_CURVE('',#6490,#6491,#1315,.T.);
#8035=EDGE_CURVE('',#6492,#6490,#1316,.T.);
#8036=EDGE_CURVE('',#6493,#6492,#1317,.T.);
#8037=EDGE_CURVE('',#6494,#6493,#1318,.T.);
#8038=EDGE_CURVE('',#6495,#6494,#1319,.T.);
#8039=EDGE_CURVE('',#6496,#6495,#1320,.T.);
#8040=EDGE_CURVE('',#6497,#6496,#1321,.T.);
#8041=EDGE_CURVE('',#6498,#6497,#1322,.T.);
#8042=EDGE_CURVE('',#6499,#6498,#1323,.T.);
#8043=EDGE_CURVE('',#6500,#6499,#1324,.T.);
#8044=EDGE_CURVE('',#6501,#6500,#1325,.T.);
#8045=EDGE_CURVE('',#6502,#6501,#1326,.T.);
#8046=EDGE_CURVE('',#6503,#6502,#1327,.T.);
#8047=EDGE_CURVE('',#6504,#6503,#1328,.T.);
#8048=EDGE_CURVE('',#6505,#6504,#1329,.T.);
#8049=EDGE_CURVE('',#6506,#6505,#1330,.T.);
#8050=EDGE_CURVE('',#6507,#6506,#1331,.T.);
#8051=EDGE_CURVE('',#6508,#6507,#1332,.T.);
#8052=EDGE_CURVE('',#6509,#6508,#1333,.T.);
#8053=EDGE_CURVE('',#6491,#6509,#1334,.T.);
#8054=EDGE_CURVE('',#6400,#6493,#1335,.T.);
#8055=EDGE_CURVE('',#6401,#6492,#1336,.T.);
#8056=EDGE_CURVE('',#6419,#6494,#1337,.T.);
#8057=EDGE_CURVE('',#6418,#6495,#1338,.T.);
#8058=EDGE_CURVE('',#6496,#6417,#1339,.T.);
#8059=EDGE_CURVE('',#6416,#6497,#1340,.T.);
#8060=EDGE_CURVE('',#6415,#6498,#1341,.T.);
#8061=EDGE_CURVE('',#6414,#6499,#1342,.T.);
#8062=EDGE_CURVE('',#6413,#6500,#1343,.T.);
#8063=EDGE_CURVE('',#6501,#6412,#1344,.T.);
#8064=EDGE_CURVE('',#6411,#6502,#1345,.T.);
#8065=EDGE_CURVE('',#6410,#6503,#1346,.T.);
#8066=EDGE_CURVE('',#6409,#6504,#1347,.T.);
#8067=EDGE_CURVE('',#6408,#6505,#1348,.T.);
#8068=EDGE_CURVE('',#6506,#6407,#1349,.T.);
#8069=EDGE_CURVE('',#6406,#6507,#1350,.T.);
#8070=EDGE_CURVE('',#6405,#6508,#1351,.T.);
#8071=EDGE_CURVE('',#6404,#6509,#1352,.T.);
#8072=EDGE_CURVE('',#6403,#6491,#1353,.T.);
#8073=EDGE_CURVE('',#6490,#6402,#1354,.T.);
#8074=EDGE_CURVE('',#6435,#6388,#747,.T.);
#8075=EDGE_CURVE('',#6432,#6386,#748,.T.);
#8076=EDGE_CURVE('',#6391,#6428,#749,.T.);
#8077=EDGE_CURVE('',#6392,#6423,#750,.T.);
#10355=ORIENTED_EDGE('',*,*,#7884,.F.);
#10356=ORIENTED_EDGE('',*,*,#7885,.T.);
#10357=ORIENTED_EDGE('',*,*,#7886,.T.);
#10358=ORIENTED_EDGE('',*,*,#7887,.T.);
#10359=ORIENTED_EDGE('',*,*,#7888,.T.);
#10360=ORIENTED_EDGE('',*,*,#7889,.F.);
#10361=ORIENTED_EDGE('',*,*,#7890,.F.);
#10362=ORIENTED_EDGE('',*,*,#7891,.F.);
#10363=ORIENTED_EDGE('',*,*,#7892,.T.);
#10364=ORIENTED_EDGE('',*,*,#7893,.T.);
#10365=ORIENTED_EDGE('',*,*,#7894,.T.);
#10366=ORIENTED_EDGE('',*,*,#7895,.T.);
#10367=ORIENTED_EDGE('',*,*,#7896,.F.);
#10368=ORIENTED_EDGE('',*,*,#7895,.F.);
#10369=ORIENTED_EDGE('',*,*,#7897,.T.);
#10370=ORIENTED_EDGE('',*,*,#7898,.T.);
#10371=ORIENTED_EDGE('',*,*,#7896,.T.);
#10372=ORIENTED_EDGE('',*,*,#7899,.T.);
#10373=ORIENTED_EDGE('',*,*,#7900,.T.);
#10374=ORIENTED_EDGE('',*,*,#7901,.T.);
#10375=ORIENTED_EDGE('',*,*,#7902,.T.);
#10376=ORIENTED_EDGE('',*,*,#7903,.T.);
#10377=ORIENTED_EDGE('',*,*,#7904,.T.);
#10378=ORIENTED_EDGE('',*,*,#7905,.T.);
#10379=ORIENTED_EDGE('',*,*,#7906,.T.);
#10380=ORIENTED_EDGE('',*,*,#7907,.T.);
#10381=ORIENTED_EDGE('',*,*,#7908,.T.);
#10382=ORIENTED_EDGE('',*,*,#7909,.T.);
#10383=ORIENTED_EDGE('',*,*,#7910,.T.);
#10384=ORIENTED_EDGE('',*,*,#7911,.T.);
#10385=ORIENTED_EDGE('',*,*,#7912,.T.);
#10386=ORIENTED_EDGE('',*,*,#7913,.T.);
#10387=ORIENTED_EDGE('',*,*,#7914,.T.);
#10388=ORIENTED_EDGE('',*,*,#7915,.T.);
#10389=ORIENTED_EDGE('',*,*,#7916,.T.);
#10390=ORIENTED_EDGE('',*,*,#7917,.T.);
#10391=ORIENTED_EDGE('',*,*,#7918,.T.);
#10392=ORIENTED_EDGE('',*,*,#7919,.T.);
#10393=ORIENTED_EDGE('',*,*,#7920,.T.);
#10394=ORIENTED_EDGE('',*,*,#7921,.F.);
#10395=ORIENTED_EDGE('',*,*,#7922,.T.);
#10396=ORIENTED_EDGE('',*,*,#7923,.T.);
#10397=ORIENTED_EDGE('',*,*,#7924,.T.);
#10398=ORIENTED_EDGE('',*,*,#7925,.T.);
#10399=ORIENTED_EDGE('',*,*,#7926,.T.);
#10400=ORIENTED_EDGE('',*,*,#7927,.F.);
#10401=ORIENTED_EDGE('',*,*,#7926,.F.);
#10402=ORIENTED_EDGE('',*,*,#7928,.T.);
#10403=ORIENTED_EDGE('',*,*,#7929,.F.);
#10404=ORIENTED_EDGE('',*,*,#7930,.F.);
#10405=ORIENTED_EDGE('',*,*,#7931,.F.);
#10406=ORIENTED_EDGE('',*,*,#7932,.F.);
#10407=ORIENTED_EDGE('',*,*,#7920,.F.);
#10408=ORIENTED_EDGE('',*,*,#7933,.T.);
#10409=ORIENTED_EDGE('',*,*,#7934,.F.);
#10410=ORIENTED_EDGE('',*,*,#7935,.F.);
#10411=ORIENTED_EDGE('',*,*,#7936,.F.);
#10412=ORIENTED_EDGE('',*,*,#7937,.F.);
#10413=ORIENTED_EDGE('',*,*,#7938,.T.);
#10414=ORIENTED_EDGE('',*,*,#7939,.T.);
#10415=ORIENTED_EDGE('',*,*,#7940,.T.);
#10416=ORIENTED_EDGE('',*,*,#7941,.F.);
#10417=ORIENTED_EDGE('',*,*,#7942,.T.);
#10418=ORIENTED_EDGE('',*,*,#7943,.T.);
#10419=ORIENTED_EDGE('',*,*,#7944,.F.);
#10420=ORIENTED_EDGE('',*,*,#7945,.F.);
#10421=ORIENTED_EDGE('',*,*,#7946,.T.);
#10422=ORIENTED_EDGE('',*,*,#7947,.T.);
#10423=ORIENTED_EDGE('',*,*,#7948,.T.);
#10424=ORIENTED_EDGE('',*,*,#7949,.T.);
#10425=ORIENTED_EDGE('',*,*,#7950,.T.);
#10426=ORIENTED_EDGE('',*,*,#7951,.T.);
#10427=ORIENTED_EDGE('',*,*,#7952,.F.);
#10428=ORIENTED_EDGE('',*,*,#7953,.F.);
#10429=ORIENTED_EDGE('',*,*,#7954,.F.);
#10430=ORIENTED_EDGE('',*,*,#7955,.F.);
#10431=ORIENTED_EDGE('',*,*,#7956,.F.);
#10432=ORIENTED_EDGE('',*,*,#7957,.T.);
#10433=ORIENTED_EDGE('',*,*,#7958,.T.);
#10434=ORIENTED_EDGE('',*,*,#7959,.T.);
#10435=ORIENTED_EDGE('',*,*,#7960,.T.);
#10436=ORIENTED_EDGE('',*,*,#7961,.T.);
#10437=ORIENTED_EDGE('',*,*,#7962,.T.);
#10438=ORIENTED_EDGE('',*,*,#7963,.T.);
#10439=ORIENTED_EDGE('',*,*,#7964,.T.);
#10440=ORIENTED_EDGE('',*,*,#7965,.T.);
#10441=ORIENTED_EDGE('',*,*,#7966,.T.);
#10442=ORIENTED_EDGE('',*,*,#7967,.T.);
#10443=ORIENTED_EDGE('',*,*,#7968,.T.);
#10444=ORIENTED_EDGE('',*,*,#7969,.T.);
#10445=ORIENTED_EDGE('',*,*,#7970,.T.);
#10446=ORIENTED_EDGE('',*,*,#7971,.T.);
#10447=ORIENTED_EDGE('',*,*,#7972,.T.);
#10448=ORIENTED_EDGE('',*,*,#7973,.T.);
#10449=ORIENTED_EDGE('',*,*,#7974,.T.);
#10450=ORIENTED_EDGE('',*,*,#7975,.T.);
#10451=ORIENTED_EDGE('',*,*,#7976,.T.);
#10452=ORIENTED_EDGE('',*,*,#7977,.T.);
#10453=ORIENTED_EDGE('',*,*,#7978,.T.);
#10454=ORIENTED_EDGE('',*,*,#7979,.T.);
#10455=ORIENTED_EDGE('',*,*,#7980,.T.);
#10456=ORIENTED_EDGE('',*,*,#7981,.T.);
#10457=ORIENTED_EDGE('',*,*,#7957,.F.);
#10458=ORIENTED_EDGE('',*,*,#7981,.F.);
#10459=ORIENTED_EDGE('',*,*,#7982,.T.);
#10460=ORIENTED_EDGE('',*,*,#7983,.T.);
#10461=ORIENTED_EDGE('',*,*,#7984,.F.);
#10462=ORIENTED_EDGE('',*,*,#7929,.T.);
#10463=ORIENTED_EDGE('',*,*,#7985,.T.);
#10464=ORIENTED_EDGE('',*,*,#7940,.F.);
#10465=ORIENTED_EDGE('',*,*,#7887,.F.);
#10466=ORIENTED_EDGE('',*,*,#7938,.F.);
#10467=ORIENTED_EDGE('',*,*,#7986,.F.);
#10468=ORIENTED_EDGE('',*,*,#7931,.T.);
#10469=ORIENTED_EDGE('',*,*,#7924,.F.);
#10470=ORIENTED_EDGE('',*,*,#7987,.T.);
#10471=ORIENTED_EDGE('',*,*,#7934,.T.);
#10472=ORIENTED_EDGE('',*,*,#7988,.T.);
#10473=ORIENTED_EDGE('',*,*,#7949,.F.);
#10474=ORIENTED_EDGE('',*,*,#7982,.F.);
#10475=ORIENTED_EDGE('',*,*,#7980,.F.);
#10476=ORIENTED_EDGE('',*,*,#7989,.F.);
#10477=ORIENTED_EDGE('',*,*,#7990,.T.);
#10478=ORIENTED_EDGE('',*,*,#7991,.F.);
#10479=ORIENTED_EDGE('',*,*,#7960,.F.);
#10480=ORIENTED_EDGE('',*,*,#7991,.T.);
#10481=ORIENTED_EDGE('',*,*,#7992,.T.);
#10482=ORIENTED_EDGE('',*,*,#7993,.F.);
#10483=ORIENTED_EDGE('',*,*,#7961,.F.);
#10484=ORIENTED_EDGE('',*,*,#7990,.F.);
#10485=ORIENTED_EDGE('',*,*,#7994,.F.);
#10486=ORIENTED_EDGE('',*,*,#7995,.F.);
#10487=ORIENTED_EDGE('',*,*,#7996,.F.);
#10488=ORIENTED_EDGE('',*,*,#7997,.F.);
#10489=ORIENTED_EDGE('',*,*,#7998,.F.);
#10490=ORIENTED_EDGE('',*,*,#7999,.F.);
#10491=ORIENTED_EDGE('',*,*,#8000,.F.);
#10492=ORIENTED_EDGE('',*,*,#8001,.F.);
#10493=ORIENTED_EDGE('',*,*,#8002,.F.);
#10494=ORIENTED_EDGE('',*,*,#8003,.F.);
#10495=ORIENTED_EDGE('',*,*,#8004,.F.);
#10496=ORIENTED_EDGE('',*,*,#8005,.F.);
#10497=ORIENTED_EDGE('',*,*,#8006,.F.);
#10498=ORIENTED_EDGE('',*,*,#8007,.F.);
#10499=ORIENTED_EDGE('',*,*,#8008,.F.);
#10500=ORIENTED_EDGE('',*,*,#8009,.F.);
#10501=ORIENTED_EDGE('',*,*,#8010,.F.);
#10502=ORIENTED_EDGE('',*,*,#8011,.F.);
#10503=ORIENTED_EDGE('',*,*,#7992,.F.);
#10504=ORIENTED_EDGE('',*,*,#8012,.T.);
#10505=ORIENTED_EDGE('',*,*,#8010,.T.);
#10506=ORIENTED_EDGE('',*,*,#8013,.F.);
#10507=ORIENTED_EDGE('',*,*,#7963,.F.);
#10508=ORIENTED_EDGE('',*,*,#8009,.T.);
#10509=ORIENTED_EDGE('',*,*,#8014,.T.);
#10510=ORIENTED_EDGE('',*,*,#7964,.F.);
#10511=ORIENTED_EDGE('',*,*,#8013,.T.);
#10512=ORIENTED_EDGE('',*,*,#8014,.F.);
#10513=ORIENTED_EDGE('',*,*,#8008,.T.);
#10514=ORIENTED_EDGE('',*,*,#8015,.F.);
#10515=ORIENTED_EDGE('',*,*,#7965,.F.);
#10516=ORIENTED_EDGE('',*,*,#8015,.T.);
#10517=ORIENTED_EDGE('',*,*,#8007,.T.);
#10518=ORIENTED_EDGE('',*,*,#8016,.F.);
#10519=ORIENTED_EDGE('',*,*,#7966,.F.);
#10520=ORIENTED_EDGE('',*,*,#7967,.F.);
#10521=ORIENTED_EDGE('',*,*,#8016,.T.);
#10522=ORIENTED_EDGE('',*,*,#8006,.T.);
#10523=ORIENTED_EDGE('',*,*,#8017,.F.);
#10524=ORIENTED_EDGE('',*,*,#8017,.T.);
#10525=ORIENTED_EDGE('',*,*,#8005,.T.);
#10526=ORIENTED_EDGE('',*,*,#8018,.F.);
#10527=ORIENTED_EDGE('',*,*,#7968,.F.);
#10528=ORIENTED_EDGE('',*,*,#8004,.T.);
#10529=ORIENTED_EDGE('',*,*,#8019,.T.);
#10530=ORIENTED_EDGE('',*,*,#7969,.F.);
#10531=ORIENTED_EDGE('',*,*,#8018,.T.);
#10532=ORIENTED_EDGE('',*,*,#8019,.F.);
#10533=ORIENTED_EDGE('',*,*,#8003,.T.);
#10534=ORIENTED_EDGE('',*,*,#8020,.F.);
#10535=ORIENTED_EDGE('',*,*,#7970,.F.);
#10536=ORIENTED_EDGE('',*,*,#8020,.T.);
#10537=ORIENTED_EDGE('',*,*,#8002,.T.);
#10538=ORIENTED_EDGE('',*,*,#8021,.F.);
#10539=ORIENTED_EDGE('',*,*,#7971,.F.);
#10540=ORIENTED_EDGE('',*,*,#7972,.F.);
#10541=ORIENTED_EDGE('',*,*,#8021,.T.);
#10542=ORIENTED_EDGE('',*,*,#8001,.T.);
#10543=ORIENTED_EDGE('',*,*,#8022,.F.);
#10544=ORIENTED_EDGE('',*,*,#8022,.T.);
#10545=ORIENTED_EDGE('',*,*,#8000,.T.);
#10546=ORIENTED_EDGE('',*,*,#8023,.F.);
#10547=ORIENTED_EDGE('',*,*,#7973,.F.);
#10548=ORIENTED_EDGE('',*,*,#7999,.T.);
#10549=ORIENTED_EDGE('',*,*,#8024,.T.);
#10550=ORIENTED_EDGE('',*,*,#7974,.F.);
#10551=ORIENTED_EDGE('',*,*,#8023,.T.);
#10552=ORIENTED_EDGE('',*,*,#8024,.F.);
#10553=ORIENTED_EDGE('',*,*,#7998,.T.);
#10554=ORIENTED_EDGE('',*,*,#8025,.F.);
#10555=ORIENTED_EDGE('',*,*,#7975,.F.);
#10556=ORIENTED_EDGE('',*,*,#8025,.T.);
#10557=ORIENTED_EDGE('',*,*,#7997,.T.);
#10558=ORIENTED_EDGE('',*,*,#8026,.F.);
#10559=ORIENTED_EDGE('',*,*,#7976,.F.);
#10560=ORIENTED_EDGE('',*,*,#7977,.F.);
#10561=ORIENTED_EDGE('',*,*,#8026,.T.);
#10562=ORIENTED_EDGE('',*,*,#7996,.T.);
#10563=ORIENTED_EDGE('',*,*,#8027,.F.);
#10564=ORIENTED_EDGE('',*,*,#8027,.T.);
#10565=ORIENTED_EDGE('',*,*,#7995,.T.);
#10566=ORIENTED_EDGE('',*,*,#8028,.F.);
#10567=ORIENTED_EDGE('',*,*,#7958,.F.);
#10568=ORIENTED_EDGE('',*,*,#7994,.T.);
#10569=ORIENTED_EDGE('',*,*,#7989,.T.);
#10570=ORIENTED_EDGE('',*,*,#7959,.F.);
#10571=ORIENTED_EDGE('',*,*,#8028,.T.);
#10572=ORIENTED_EDGE('',*,*,#7962,.F.);
#10573=ORIENTED_EDGE('',*,*,#7993,.T.);
#10574=ORIENTED_EDGE('',*,*,#8011,.T.);
#10575=ORIENTED_EDGE('',*,*,#8012,.F.);
#10576=ORIENTED_EDGE('',*,*,#7978,.F.);
#10577=ORIENTED_EDGE('',*,*,#7953,.T.);
#10578=ORIENTED_EDGE('',*,*,#7979,.F.);
#10579=ORIENTED_EDGE('',*,*,#7952,.T.);
#10580=ORIENTED_EDGE('',*,*,#8029,.T.);
#10581=ORIENTED_EDGE('',*,*,#7950,.F.);
#10582=ORIENTED_EDGE('',*,*,#7983,.F.);
#10583=ORIENTED_EDGE('',*,*,#7948,.F.);
#10584=ORIENTED_EDGE('',*,*,#7893,.F.);
#10585=ORIENTED_EDGE('',*,*,#7954,.T.);
#10586=ORIENTED_EDGE('',*,*,#7919,.F.);
#10587=ORIENTED_EDGE('',*,*,#7937,.T.);
#10588=ORIENTED_EDGE('',*,*,#8030,.T.);
#10589=ORIENTED_EDGE('',*,*,#7921,.T.);
#10590=ORIENTED_EDGE('',*,*,#7932,.T.);
#10591=ORIENTED_EDGE('',*,*,#7986,.T.);
#10592=ORIENTED_EDGE('',*,*,#8029,.F.);
#10593=ORIENTED_EDGE('',*,*,#7951,.F.);
#10594=ORIENTED_EDGE('',*,*,#7927,.T.);
#10595=ORIENTED_EDGE('',*,*,#7898,.F.);
#10596=ORIENTED_EDGE('',*,*,#7946,.F.);
#10597=ORIENTED_EDGE('',*,*,#8031,.F.);
#10598=ORIENTED_EDGE('',*,*,#7956,.T.);
#10599=ORIENTED_EDGE('',*,*,#7945,.T.);
#10600=ORIENTED_EDGE('',*,*,#8031,.T.);
#10601=ORIENTED_EDGE('',*,*,#7925,.F.);
#10602=ORIENTED_EDGE('',*,*,#7988,.F.);
#10603=ORIENTED_EDGE('',*,*,#7933,.F.);
#10604=ORIENTED_EDGE('',*,*,#7985,.F.);
#10605=ORIENTED_EDGE('',*,*,#7928,.F.);
#10606=ORIENTED_EDGE('',*,*,#8032,.F.);
#10607=ORIENTED_EDGE('',*,*,#7943,.F.);
#10608=ORIENTED_EDGE('',*,*,#8032,.T.);
#10609=ORIENTED_EDGE('',*,*,#7942,.F.);
#10610=ORIENTED_EDGE('',*,*,#8033,.F.);
#10611=ORIENTED_EDGE('',*,*,#7944,.T.);
#10612=ORIENTED_EDGE('',*,*,#7941,.T.);
#10613=ORIENTED_EDGE('',*,*,#8033,.T.);
#10614=ORIENTED_EDGE('',*,*,#7936,.T.);
#10615=ORIENTED_EDGE('',*,*,#7891,.T.);
#10616=ORIENTED_EDGE('',*,*,#7922,.F.);
#10617=ORIENTED_EDGE('',*,*,#8030,.F.);
#10618=ORIENTED_EDGE('',*,*,#8034,.F.);
#10619=ORIENTED_EDGE('',*,*,#8035,.F.);
#10620=ORIENTED_EDGE('',*,*,#8036,.F.);
#10621=ORIENTED_EDGE('',*,*,#8037,.F.);
#10622=ORIENTED_EDGE('',*,*,#8038,.F.);
#10623=ORIENTED_EDGE('',*,*,#8039,.F.);
#10624=ORIENTED_EDGE('',*,*,#8040,.F.);
#10625=ORIENTED_EDGE('',*,*,#8041,.F.);
#10626=ORIENTED_EDGE('',*,*,#8042,.F.);
#10627=ORIENTED_EDGE('',*,*,#8043,.F.);
#10628=ORIENTED_EDGE('',*,*,#8044,.F.);
#10629=ORIENTED_EDGE('',*,*,#8045,.F.);
#10630=ORIENTED_EDGE('',*,*,#8046,.F.);
#10631=ORIENTED_EDGE('',*,*,#8047,.F.);
#10632=ORIENTED_EDGE('',*,*,#8048,.F.);
#10633=ORIENTED_EDGE('',*,*,#8049,.F.);
#10634=ORIENTED_EDGE('',*,*,#8050,.F.);
#10635=ORIENTED_EDGE('',*,*,#8051,.F.);
#10636=ORIENTED_EDGE('',*,*,#8052,.F.);
#10637=ORIENTED_EDGE('',*,*,#8053,.F.);
#10638=ORIENTED_EDGE('',*,*,#8054,.T.);
#10639=ORIENTED_EDGE('',*,*,#8036,.T.);
#10640=ORIENTED_EDGE('',*,*,#8055,.F.);
#10641=ORIENTED_EDGE('',*,*,#7899,.F.);
#10642=ORIENTED_EDGE('',*,*,#7918,.F.);
#10643=ORIENTED_EDGE('',*,*,#8056,.T.);
#10644=ORIENTED_EDGE('',*,*,#8037,.T.);
#10645=ORIENTED_EDGE('',*,*,#8054,.F.);
#10646=ORIENTED_EDGE('',*,*,#8057,.T.);
#10647=ORIENTED_EDGE('',*,*,#8038,.T.);
#10648=ORIENTED_EDGE('',*,*,#8056,.F.);
#10649=ORIENTED_EDGE('',*,*,#7917,.F.);
#10650=ORIENTED_EDGE('',*,*,#8058,.F.);
#10651=ORIENTED_EDGE('',*,*,#8039,.T.);
#10652=ORIENTED_EDGE('',*,*,#8057,.F.);
#10653=ORIENTED_EDGE('',*,*,#7916,.F.);
#10654=ORIENTED_EDGE('',*,*,#8040,.T.);
#10655=ORIENTED_EDGE('',*,*,#8058,.T.);
#10656=ORIENTED_EDGE('',*,*,#7915,.F.);
#10657=ORIENTED_EDGE('',*,*,#8059,.T.);
#10658=ORIENTED_EDGE('',*,*,#8060,.T.);
#10659=ORIENTED_EDGE('',*,*,#8041,.T.);
#10660=ORIENTED_EDGE('',*,*,#8059,.F.);
#10661=ORIENTED_EDGE('',*,*,#7914,.F.);
#10662=ORIENTED_EDGE('',*,*,#7913,.F.);
#10663=ORIENTED_EDGE('',*,*,#8061,.T.);
#10664=ORIENTED_EDGE('',*,*,#8042,.T.);
#10665=ORIENTED_EDGE('',*,*,#8060,.F.);
#10666=ORIENTED_EDGE('',*,*,#8062,.T.);
#10667=ORIENTED_EDGE('',*,*,#8043,.T.);
#10668=ORIENTED_EDGE('',*,*,#8061,.F.);
#10669=ORIENTED_EDGE('',*,*,#7912,.F.);
#10670=ORIENTED_EDGE('',*,*,#8063,.F.);
#10671=ORIENTED_EDGE('',*,*,#8044,.T.);
#10672=ORIENTED_EDGE('',*,*,#8062,.F.);
#10673=ORIENTED_EDGE('',*,*,#7911,.F.);
#10674=ORIENTED_EDGE('',*,*,#8045,.T.);
#10675=ORIENTED_EDGE('',*,*,#8063,.T.);
#10676=ORIENTED_EDGE('',*,*,#7910,.F.);
#10677=ORIENTED_EDGE('',*,*,#8064,.T.);
#10678=ORIENTED_EDGE('',*,*,#8065,.T.);
#10679=ORIENTED_EDGE('',*,*,#8046,.T.);
#10680=ORIENTED_EDGE('',*,*,#8064,.F.);
#10681=ORIENTED_EDGE('',*,*,#7909,.F.);
#10682=ORIENTED_EDGE('',*,*,#7908,.F.);
#10683=ORIENTED_EDGE('',*,*,#8066,.T.);
#10684=ORIENTED_EDGE('',*,*,#8047,.T.);
#10685=ORIENTED_EDGE('',*,*,#8065,.F.);
#10686=ORIENTED_EDGE('',*,*,#8067,.T.);
#10687=ORIENTED_EDGE('',*,*,#8048,.T.);
#10688=ORIENTED_EDGE('',*,*,#8066,.F.);
#10689=ORIENTED_EDGE('',*,*,#7907,.F.);
#10690=ORIENTED_EDGE('',*,*,#8068,.F.);
#10691=ORIENTED_EDGE('',*,*,#8049,.T.);
#10692=ORIENTED_EDGE('',*,*,#8067,.F.);
#10693=ORIENTED_EDGE('',*,*,#7906,.F.);
#10694=ORIENTED_EDGE('',*,*,#8050,.T.);
#10695=ORIENTED_EDGE('',*,*,#8068,.T.);
#10696=ORIENTED_EDGE('',*,*,#7905,.F.);
#10697=ORIENTED_EDGE('',*,*,#8069,.T.);
#10698=ORIENTED_EDGE('',*,*,#8070,.T.);
#10699=ORIENTED_EDGE('',*,*,#8051,.T.);
#10700=ORIENTED_EDGE('',*,*,#8069,.F.);
#10701=ORIENTED_EDGE('',*,*,#7904,.F.);
#10702=ORIENTED_EDGE('',*,*,#7903,.F.);
#10703=ORIENTED_EDGE('',*,*,#8071,.T.);
#10704=ORIENTED_EDGE('',*,*,#8052,.T.);
#10705=ORIENTED_EDGE('',*,*,#8070,.F.);
#10706=ORIENTED_EDGE('',*,*,#8072,.T.);
#10707=ORIENTED_EDGE('',*,*,#8053,.T.);
#10708=ORIENTED_EDGE('',*,*,#8071,.F.);
#10709=ORIENTED_EDGE('',*,*,#7902,.F.);
#10710=ORIENTED_EDGE('',*,*,#8073,.F.);
#10711=ORIENTED_EDGE('',*,*,#8034,.T.);
#10712=ORIENTED_EDGE('',*,*,#8072,.F.);
#10713=ORIENTED_EDGE('',*,*,#7901,.F.);
#10714=ORIENTED_EDGE('',*,*,#8035,.T.);
#10715=ORIENTED_EDGE('',*,*,#8073,.T.);
#10716=ORIENTED_EDGE('',*,*,#7900,.F.);
#10717=ORIENTED_EDGE('',*,*,#8055,.T.);
#10718=ORIENTED_EDGE('',*,*,#7892,.F.);
#10719=ORIENTED_EDGE('',*,*,#7955,.T.);
#10720=ORIENTED_EDGE('',*,*,#7947,.F.);
#10721=ORIENTED_EDGE('',*,*,#7897,.F.);
#10722=ORIENTED_EDGE('',*,*,#7894,.F.);
#10723=ORIENTED_EDGE('',*,*,#7939,.F.);
#10724=ORIENTED_EDGE('',*,*,#7886,.F.);
#10725=ORIENTED_EDGE('',*,*,#8074,.F.);
#10726=ORIENTED_EDGE('',*,*,#8075,.T.);
#10727=ORIENTED_EDGE('',*,*,#7884,.T.);
#10728=ORIENTED_EDGE('',*,*,#7935,.T.);
#10729=ORIENTED_EDGE('',*,*,#7888,.F.);
#10730=ORIENTED_EDGE('',*,*,#7930,.T.);
#10731=ORIENTED_EDGE('',*,*,#8076,.F.);
#10732=ORIENTED_EDGE('',*,*,#7885,.F.);
#10733=ORIENTED_EDGE('',*,*,#8075,.F.);
#10734=ORIENTED_EDGE('',*,*,#7987,.F.);
#10735=ORIENTED_EDGE('',*,*,#8077,.F.);
#10736=ORIENTED_EDGE('',*,*,#7889,.T.);
#10737=ORIENTED_EDGE('',*,*,#8076,.T.);
#10738=ORIENTED_EDGE('',*,*,#7984,.T.);
#10739=ORIENTED_EDGE('',*,*,#8074,.T.);
#10740=ORIENTED_EDGE('',*,*,#7923,.F.);
#10741=ORIENTED_EDGE('',*,*,#7890,.T.);
#10742=ORIENTED_EDGE('',*,*,#8077,.T.);
#14441=ADVANCED_FACE('',(#3806),#147,.F.);
#14442=ADVANCED_FACE('',(#3807),#3461,.T.);
#14443=ADVANCED_FACE('',(#3808,#212),#80,.T.);
#14444=ADVANCED_FACE('',(#3809,#213,#214,#215),#3462,.T.);
#14445=ADVANCED_FACE('',(#3810,#216),#81,.T.);
#14446=ADVANCED_FACE('',(#3811),#3463,.T.);
#14447=ADVANCED_FACE('',(#3812),#365,.F.);
#14448=ADVANCED_FACE('',(#3813),#366,.F.);
#14449=ADVANCED_FACE('',(#3814),#367,.F.);
#14450=ADVANCED_FACE('',(#3815),#368,.T.);
#14451=ADVANCED_FACE('',(#3816),#369,.F.);
#14452=ADVANCED_FACE('',(#3817),#370,.F.);
#14453=ADVANCED_FACE('',(#3818),#371,.F.);
#14454=ADVANCED_FACE('',(#3819),#372,.F.);
#14455=ADVANCED_FACE('',(#3820),#373,.F.);
#14456=ADVANCED_FACE('',(#3821),#374,.F.);
#14457=ADVANCED_FACE('',(#3822),#375,.F.);
#14458=ADVANCED_FACE('',(#3823),#376,.F.);
#14459=ADVANCED_FACE('',(#3824),#377,.F.);
#14460=ADVANCED_FACE('',(#3825),#378,.F.);
#14461=ADVANCED_FACE('',(#3826),#379,.F.);
#14462=ADVANCED_FACE('',(#3827),#380,.F.);
#14463=ADVANCED_FACE('',(#3828),#381,.F.);
#14464=ADVANCED_FACE('',(#3829),#382,.F.);
#14465=ADVANCED_FACE('',(#3830),#383,.F.);
#14466=ADVANCED_FACE('',(#3831),#384,.F.);
#14467=ADVANCED_FACE('',(#3832),#385,.F.);
#14468=ADVANCED_FACE('',(#3833),#386,.F.);
#14469=ADVANCED_FACE('',(#3834),#387,.F.);
#14470=ADVANCED_FACE('',(#3835),#388,.F.);
#14471=ADVANCED_FACE('',(#3836),#389,.F.);
#14472=ADVANCED_FACE('',(#3837),#390,.T.);
#14473=ADVANCED_FACE('',(#3838),#391,.F.);
#14474=ADVANCED_FACE('',(#3839),#392,.F.);
#14475=ADVANCED_FACE('',(#3840),#393,.F.);
#14476=ADVANCED_FACE('',(#3841),#394,.F.);
#14477=ADVANCED_FACE('',(#3842),#395,.T.);
#14478=ADVANCED_FACE('',(#3843),#396,.T.);
#14479=ADVANCED_FACE('',(#3844),#397,.F.);
#14480=ADVANCED_FACE('',(#3845),#398,.F.);
#14481=ADVANCED_FACE('',(#3846),#399,.T.);
#14482=ADVANCED_FACE('',(#3847),#400,.T.);
#14483=ADVANCED_FACE('',(#3848),#401,.F.);
#14484=ADVANCED_FACE('',(#3849),#402,.F.);
#14485=ADVANCED_FACE('',(#3850),#403,.F.);
#14486=ADVANCED_FACE('',(#3851),#404,.F.);
#14487=ADVANCED_FACE('',(#3852),#405,.F.);
#14488=ADVANCED_FACE('',(#3853),#406,.F.);
#14489=ADVANCED_FACE('',(#3854),#407,.F.);
#14490=ADVANCED_FACE('',(#3855),#408,.F.);
#14491=ADVANCED_FACE('',(#3856),#409,.F.);
#14492=ADVANCED_FACE('',(#3857),#410,.F.);
#14493=ADVANCED_FACE('',(#3858),#411,.F.);
#14494=ADVANCED_FACE('',(#3859),#412,.F.);
#14495=ADVANCED_FACE('',(#3860),#413,.F.);
#14496=ADVANCED_FACE('',(#3861),#414,.F.);
#14497=ADVANCED_FACE('',(#3862),#415,.F.);
#14498=ADVANCED_FACE('',(#3863),#416,.F.);
#14499=ADVANCED_FACE('',(#3864),#417,.F.);
#14500=ADVANCED_FACE('',(#3865),#418,.F.);
#14501=ADVANCED_FACE('',(#3866),#419,.F.);
#14502=ADVANCED_FACE('',(#3867),#420,.F.);
#14503=ADVANCED_FACE('',(#3868),#421,.F.);
#14504=ADVANCED_FACE('',(#3869),#422,.F.);
#14505=ADVANCED_FACE('',(#3870),#423,.F.);
#14506=ADVANCED_FACE('',(#3871),#424,.F.);
#14507=ADVANCED_FACE('',(#3872),#425,.T.);
#14508=ADVANCED_FACE('',(#3873),#426,.T.);
#14509=ADVANCED_FACE('',(#3874),#427,.F.);
#14510=ADVANCED_FACE('',(#3875),#428,.T.);
#14511=ADVANCED_FACE('',(#3876),#429,.F.);
#14512=ADVANCED_FACE('',(#3877),#148,.F.);
#14513=ADVANCED_FACE('',(#3878),#430,.T.);
#15194=CLOSED_SHELL('',(#14441,#14442,#14443,#14444,#14445,#14446,#14447,
#14448,#14449,#14450,#14451,#14452,#14453,#14454,#14455,#14456,#14457,#14458,
#14459,#14460,#14461,#14462,#14463,#14464,#14465,#14466,#14467,#14468,#14469,
#14470,#14471,#14472,#14473,#14474,#14475,#14476,#14477,#14478,#14479,#14480,
#14481,#14482,#14483,#14484,#14485,#14486,#14487,#14488,#14489,#14490,#14491,
#14492,#14493,#14494,#14495,#14496,#14497,#14498,#14499,#14500,#14501,#14502,
#14503,#14504,#14505,#14506,#14507,#14508,#14509,#14510,#14511,#14512,#14513));
#15531=AXIS2_PLACEMENT_3D('',#34069,#17524,#17525);
#15532=AXIS2_PLACEMENT_3D('',#34080,#17526,#17527);
#15533=AXIS2_PLACEMENT_3D('',#34084,#17529,#17530);
#15534=AXIS2_PLACEMENT_3D('',#34086,#17531,#17532);
#15535=AXIS2_PLACEMENT_3D('',#34088,#17533,#17534);
#15536=AXIS2_PLACEMENT_3D('',#34092,#17536,#17537);
#15537=AXIS2_PLACEMENT_3D('',#34093,#17538,#17539);
#15538=AXIS2_PLACEMENT_3D('',#34094,#17540,#17541);
#15539=AXIS2_PLACEMENT_3D('',#34097,#17542,#17543);
#15540=AXIS2_PLACEMENT_3D('',#34099,#17544,#17545);
#15541=AXIS2_PLACEMENT_3D('',#34101,#17546,#17547);
#15542=AXIS2_PLACEMENT_3D('',#34104,#17549,#17550);
#15543=AXIS2_PLACEMENT_3D('',#34106,#17551,#17552);
#15544=AXIS2_PLACEMENT_3D('',#34107,#17553,#17554);
#15545=AXIS2_PLACEMENT_3D('',#34108,#17555,#17556);
#15546=AXIS2_PLACEMENT_3D('',#34111,#17557,#17558);
#15547=AXIS2_PLACEMENT_3D('',#34113,#17559,#17560);
#15548=AXIS2_PLACEMENT_3D('',#34115,#17561,#17562);
#15549=AXIS2_PLACEMENT_3D('',#34117,#17563,#17564);
#15550=AXIS2_PLACEMENT_3D('',#34119,#17565,#17566);
#15551=AXIS2_PLACEMENT_3D('',#34121,#17567,#17568);
#15552=AXIS2_PLACEMENT_3D('',#34123,#17569,#17570);
#15553=AXIS2_PLACEMENT_3D('',#34125,#17571,#17572);
#15554=AXIS2_PLACEMENT_3D('',#34127,#17573,#17574);
#15555=AXIS2_PLACEMENT_3D('',#34129,#17575,#17576);
#15556=AXIS2_PLACEMENT_3D('',#34131,#17577,#17578);
#15557=AXIS2_PLACEMENT_3D('',#34133,#17579,#17580);
#15558=AXIS2_PLACEMENT_3D('',#34135,#17581,#17582);
#15559=AXIS2_PLACEMENT_3D('',#34137,#17583,#17584);
#15560=AXIS2_PLACEMENT_3D('',#34139,#17585,#17586);
#15561=AXIS2_PLACEMENT_3D('',#34141,#17587,#17588);
#15562=AXIS2_PLACEMENT_3D('',#34143,#17589,#17590);
#15563=AXIS2_PLACEMENT_3D('',#34145,#17591,#17592);
#15564=AXIS2_PLACEMENT_3D('',#34147,#17593,#17594);
#15565=AXIS2_PLACEMENT_3D('',#34148,#17595,#17596);
#15566=AXIS2_PLACEMENT_3D('',#34149,#17597,#17598);
#15567=AXIS2_PLACEMENT_3D('',#34151,#17599,#17600);
#15568=AXIS2_PLACEMENT_3D('',#34155,#17602,#17603);
#15569=AXIS2_PLACEMENT_3D('',#34162,#17607,#17608);
#15570=AXIS2_PLACEMENT_3D('',#34165,#17610,#17611);
#15571=AXIS2_PLACEMENT_3D('',#34167,#17612,#17613);
#15572=AXIS2_PLACEMENT_3D('',#34173,#17617,#17618);
#15573=AXIS2_PLACEMENT_3D('',#34176,#17619,#17620);
#15574=AXIS2_PLACEMENT_3D('',#34183,#17624,#17625);
#15575=AXIS2_PLACEMENT_3D('',#34190,#17629,#17630);
#15576=AXIS2_PLACEMENT_3D('',#34194,#17632,#17633);
#15577=AXIS2_PLACEMENT_3D('',#34198,#17635,#17636);
#15578=AXIS2_PLACEMENT_3D('',#34208,#17642,#17643);
#15579=AXIS2_PLACEMENT_3D('',#34216,#17649,#17650);
#15580=AXIS2_PLACEMENT_3D('',#34218,#17651,#17652);
#15581=AXIS2_PLACEMENT_3D('',#34221,#17653,#17654);
#15582=AXIS2_PLACEMENT_3D('',#34223,#17655,#17656);
#15583=AXIS2_PLACEMENT_3D('',#34225,#17657,#17658);
#15584=AXIS2_PLACEMENT_3D('',#34227,#17659,#17660);
#15585=AXIS2_PLACEMENT_3D('',#34229,#17661,#17662);
#15586=AXIS2_PLACEMENT_3D('',#34231,#17663,#17664);
#15587=AXIS2_PLACEMENT_3D('',#34233,#17665,#17666);
#15588=AXIS2_PLACEMENT_3D('',#34235,#17667,#17668);
#15589=AXIS2_PLACEMENT_3D('',#34237,#17669,#17670);
#15590=AXIS2_PLACEMENT_3D('',#34239,#17671,#17672);
#15591=AXIS2_PLACEMENT_3D('',#34241,#17673,#17674);
#15592=AXIS2_PLACEMENT_3D('',#34243,#17675,#17676);
#15593=AXIS2_PLACEMENT_3D('',#34245,#17677,#17678);
#15594=AXIS2_PLACEMENT_3D('',#34247,#17679,#17680);
#15595=AXIS2_PLACEMENT_3D('',#34249,#17681,#17682);
#15596=AXIS2_PLACEMENT_3D('',#34251,#17683,#17684);
#15597=AXIS2_PLACEMENT_3D('',#34253,#17685,#17686);
#15598=AXIS2_PLACEMENT_3D('',#34255,#17687,#17688);
#15599=AXIS2_PLACEMENT_3D('',#34257,#17689,#17690);
#15600=AXIS2_PLACEMENT_3D('',#34258,#17691,#17692);
#15601=AXIS2_PLACEMENT_3D('',#34259,#17693,#17694);
#15602=AXIS2_PLACEMENT_3D('',#34260,#17695,#17696);
#15603=AXIS2_PLACEMENT_3D('',#34261,#17697,#17698);
#15604=AXIS2_PLACEMENT_3D('',#34263,#17699,#17700);
#15605=AXIS2_PLACEMENT_3D('',#34265,#17702,#17703);
#15606=AXIS2_PLACEMENT_3D('',#34266,#17704,#17705);
#15607=AXIS2_PLACEMENT_3D('',#34267,#17706,#17707);
#15608=AXIS2_PLACEMENT_3D('',#34268,#17708,#17709);
#15609=AXIS2_PLACEMENT_3D('',#34270,#17711,#17712);
#15610=AXIS2_PLACEMENT_3D('',#34272,#17714,#17715);
#15611=AXIS2_PLACEMENT_3D('',#34273,#17716,#17717);
#15612=AXIS2_PLACEMENT_3D('',#34275,#17719,#17720);
#15613=AXIS2_PLACEMENT_3D('',#34276,#17721,#17722);
#15614=AXIS2_PLACEMENT_3D('',#34282,#17726,#17727);
#15615=AXIS2_PLACEMENT_3D('',#34286,#17730,#17731);
#15616=AXIS2_PLACEMENT_3D('',#34322,#17750,#17751);
#15617=AXIS2_PLACEMENT_3D('',#34325,#17754,#17755);
#15618=AXIS2_PLACEMENT_3D('',#34327,#17757,#17758);
#15619=AXIS2_PLACEMENT_3D('',#34329,#17760,#17761);
#15620=AXIS2_PLACEMENT_3D('',#34331,#17763,#17764);
#15621=AXIS2_PLACEMENT_3D('',#34333,#17766,#17767);
#15622=AXIS2_PLACEMENT_3D('',#34335,#17769,#17770);
#15623=AXIS2_PLACEMENT_3D('',#34337,#17772,#17773);
#15624=AXIS2_PLACEMENT_3D('',#34339,#17775,#17776);
#15625=AXIS2_PLACEMENT_3D('',#34341,#17778,#17779);
#15626=AXIS2_PLACEMENT_3D('',#34343,#17781,#17782);
#15627=AXIS2_PLACEMENT_3D('',#34345,#17784,#17785);
#15628=AXIS2_PLACEMENT_3D('',#34347,#17787,#17788);
#15629=AXIS2_PLACEMENT_3D('',#34349,#17790,#17791);
#15630=AXIS2_PLACEMENT_3D('',#34351,#17793,#17794);
#15631=AXIS2_PLACEMENT_3D('',#34353,#17796,#17797);
#15632=AXIS2_PLACEMENT_3D('',#34355,#17799,#17800);
#15633=AXIS2_PLACEMENT_3D('',#34356,#17801,#17802);
#15634=AXIS2_PLACEMENT_3D('',#34357,#17803,#17804);
#15635=AXIS2_PLACEMENT_3D('',#34358,#17805,#17806);
#15636=AXIS2_PLACEMENT_3D('',#34360,#17808,#17809);
#15637=AXIS2_PLACEMENT_3D('',#34361,#17810,#17811);
#15638=AXIS2_PLACEMENT_3D('',#34362,#17812,#17813);
#15639=AXIS2_PLACEMENT_3D('',#34364,#17815,#17816);
#15640=AXIS2_PLACEMENT_3D('',#34365,#17817,#17818);
#15641=AXIS2_PLACEMENT_3D('',#34366,#17819,#17820);
#15642=AXIS2_PLACEMENT_3D('',#34368,#17822,#17823);
#15643=AXIS2_PLACEMENT_3D('',#34369,#17824,#17825);
#15644=AXIS2_PLACEMENT_3D('',#34370,#17826,#17827);
#15645=AXIS2_PLACEMENT_3D('',#34372,#17829,#17830);
#15646=AXIS2_PLACEMENT_3D('',#34374,#17832,#17833);
#15647=AXIS2_PLACEMENT_3D('',#34375,#17834,#17835);
#15648=AXIS2_PLACEMENT_3D('',#34376,#17836,#17837);
#15649=AXIS2_PLACEMENT_3D('',#34417,#17858,#17859);
#15650=AXIS2_PLACEMENT_3D('',#34420,#17862,#17863);
#15651=AXIS2_PLACEMENT_3D('',#34422,#17865,#17866);
#15652=AXIS2_PLACEMENT_3D('',#34424,#17868,#17869);
#15653=AXIS2_PLACEMENT_3D('',#34426,#17871,#17872);
#15654=AXIS2_PLACEMENT_3D('',#34428,#17874,#17875);
#15655=AXIS2_PLACEMENT_3D('',#34430,#17877,#17878);
#15656=AXIS2_PLACEMENT_3D('',#34432,#17880,#17881);
#15657=AXIS2_PLACEMENT_3D('',#34434,#17883,#17884);
#15658=AXIS2_PLACEMENT_3D('',#34436,#17886,#17887);
#15659=AXIS2_PLACEMENT_3D('',#34438,#17889,#17890);
#15660=AXIS2_PLACEMENT_3D('',#34440,#17892,#17893);
#15661=AXIS2_PLACEMENT_3D('',#34442,#17895,#17896);
#15662=AXIS2_PLACEMENT_3D('',#34444,#17898,#17899);
#15663=AXIS2_PLACEMENT_3D('',#34446,#17901,#17902);
#15664=AXIS2_PLACEMENT_3D('',#34448,#17904,#17905);
#15665=AXIS2_PLACEMENT_3D('',#34450,#17907,#17908);
#15666=AXIS2_PLACEMENT_3D('',#34452,#17910,#17911);
#15667=AXIS2_PLACEMENT_3D('',#34454,#17913,#17914);
#15668=AXIS2_PLACEMENT_3D('',#34456,#17916,#17917);
#15669=AXIS2_PLACEMENT_3D('',#34457,#17918,#17919);
#15670=AXIS2_PLACEMENT_3D('',#34458,#17920,#17921);
#15671=AXIS2_PLACEMENT_3D('',#34459,#17922,#17923);
#15672=AXIS2_PLACEMENT_3D('',#34460,#17924,#17925);
#15673=AXIS2_PLACEMENT_3D('',#34461,#17926,#17927);
#15674=AXIS2_PLACEMENT_3D('',#34462,#17928,#17929);
#15675=AXIS2_PLACEMENT_3D('',#34463,#17930,#17931);
#15676=AXIS2_PLACEMENT_3D('',#34464,#17932,#17933);
#15677=AXIS2_PLACEMENT_3D('',#34473,#17934,#17935);
#15678=AXIS2_PLACEMENT_3D('',#34474,#17936,#17937);
#17524=DIRECTION('axis',(0.,0.,1.));
#17525=DIRECTION('refdir',(1.,0.,0.));
#17526=DIRECTION('center_axis',(3.88843322550999E-16,0.978147600733806,
-0.207911690817759));
#17527=DIRECTION('ref_axis',(-5.50265365050884E-13,0.207911690817759,0.978147600733806));
#17528=DIRECTION('',(0.,-0.978147600733805,0.20791169081776));
#17529=DIRECTION('center_axis',(-3.43097049309705E-16,0.978147600733805,
-0.20791169081776));
#17530=DIRECTION('ref_axis',(3.33622364636221E-13,0.20791169081776,0.978147600733805));
#17531=DIRECTION('center_axis',(2.9543986082272E-15,0.978147600733806,-0.20791169081776));
#17532=DIRECTION('ref_axis',(1.67939778347642E-14,0.20791169081776,0.978147600733806));
#17533=DIRECTION('center_axis',(-9.14925464825879E-17,0.978147600733805,
-0.20791169081776));
#17534=DIRECTION('ref_axis',(-7.57549072892314E-14,0.20791169081776,0.978147600733805));
#17535=DIRECTION('',(0.,-0.978147600733805,0.20791169081776));
#17536=DIRECTION('center_axis',(-6.86194098619411E-16,0.978147600733806,
-0.207911690817759));
#17537=DIRECTION('ref_axis',(-2.36047899524434E-14,0.207911690817759,0.978147600733806));
#17538=DIRECTION('center_axis',(-1.85321367243343E-14,0.978147600733805,
-0.207911690817761));
#17539=DIRECTION('ref_axis',(4.13512095738825E-13,0.207911690817761,0.978147600733805));
#17540=DIRECTION('center_axis',(1.E-15,0.978147600733805,-0.20791169081776));
#17541=DIRECTION('ref_axis',(2.24944215683689E-31,0.20791169081776,0.978147600733806));
#17542=DIRECTION('center_axis',(-1.E-15,-0.978147600733805,0.20791169081776));
#17543=DIRECTION('ref_axis',(2.00292312395533E-31,0.20791169081776,0.978147600733806));
#17544=DIRECTION('center_axis',(-1.E-15,-0.978147600733805,0.20791169081776));
#17545=DIRECTION('ref_axis',(2.00292312395533E-31,0.20791169081776,0.978147600733806));
#17546=DIRECTION('center_axis',(-1.E-15,-0.978147600733805,0.20791169081776));
#17547=DIRECTION('ref_axis',(2.00292312395533E-31,0.20791169081776,0.978147600733806));
#17548=DIRECTION('',(-1.E-15,-0.978147600733806,0.20791169081776));
#17549=DIRECTION('center_axis',(-1.E-15,-0.978147600733805,0.20791169081776));
#17550=DIRECTION('ref_axis',(2.00292312395533E-31,0.20791169081776,0.978147600733806));
#17551=DIRECTION('center_axis',(-1.E-15,-0.978147600733805,0.20791169081776));
#17552=DIRECTION('ref_axis',(2.00292312395533E-31,0.20791169081776,0.978147600733806));
#17553=DIRECTION('center_axis',(-1.E-15,-0.978147600733805,0.20791169081776));
#17554=DIRECTION('ref_axis',(2.00292312395533E-31,0.20791169081776,0.978147600733806));
#17555=DIRECTION('center_axis',(-1.48029736616688E-16,-0.20791169081776,
-0.978147600733806));
#17556=DIRECTION('ref_axis',(-1.,1.1842378929335E-15,-2.08166817117217E-16));
#17557=DIRECTION('center_axis',(-1.,9.78147600733805E-16,-2.0791169081776E-16));
#17558=DIRECTION('ref_axis',(-3.70646524662632E-31,0.20791169081776,0.978147600733806));
#17559=DIRECTION('center_axis',(0.,0.20791169081776,0.978147600733805));
#17560=DIRECTION('ref_axis',(1.01403901935241E-15,0.978147600733806,-0.20791169081776));
#17561=DIRECTION('center_axis',(-0.824041924199368,-0.117787965463444,-0.55414880885353));
#17562=DIRECTION('ref_axis',(-0.566528822887065,0.171327949765011,0.80603463105968));
#17563=DIRECTION('center_axis',(0.566528822887065,0.171327949765011,0.80603463105968));
#17564=DIRECTION('ref_axis',(0.824041924199368,-0.117787965463446,-0.554148808853529));
#17565=DIRECTION('center_axis',(-1.,9.78147600733805E-16,-2.0791169081776E-16));
#17566=DIRECTION('ref_axis',(-7.79618225341413E-32,0.20791169081776,0.978147600733805));
#17567=DIRECTION('center_axis',(0.,0.20791169081776,0.978147600733805));
#17568=DIRECTION('ref_axis',(1.04747777942724E-15,0.978147600733805,-0.20791169081776));
#17569=DIRECTION('center_axis',(1.,-9.78147600733805E-16,2.0791169081776E-16));
#17570=DIRECTION('ref_axis',(4.19950331238945E-31,-0.20791169081776,-0.978147600733806));
#17571=DIRECTION('center_axis',(-0.566528822887065,0.171327949765012,0.80603463105968));
#17572=DIRECTION('ref_axis',(0.824041924199368,0.117787965463444,0.55414880885353));
#17573=DIRECTION('center_axis',(0.824041924199368,-0.117787965463446,-0.554148808853529));
#17574=DIRECTION('ref_axis',(-0.566528822887065,-0.17132794976501,-0.80603463105968));
#17575=DIRECTION('center_axis',(0.,0.20791169081776,0.978147600733805));
#17576=DIRECTION('ref_axis',(1.01403901935241E-15,0.978147600733806,-0.20791169081776));
#17577=DIRECTION('center_axis',(1.,-9.78147600733805E-16,2.0791169081776E-16));
#17578=DIRECTION('ref_axis',(2.21166036268998E-31,-0.20791169081776,-0.978147600733805));
#17579=DIRECTION('center_axis',(0.,-0.20791169081776,-0.978147600733805));
#17580=DIRECTION('ref_axis',(-1.01403901935241E-15,-0.978147600733806,0.20791169081776));
#17581=DIRECTION('center_axis',(0.824041924199368,0.117787965463444,0.55414880885353));
#17582=DIRECTION('ref_axis',(0.566528822887065,-0.171327949765011,-0.80603463105968));
#17583=DIRECTION('center_axis',(-0.566528822887065,-0.171327949765011,-0.80603463105968));
#17584=DIRECTION('ref_axis',(-0.824041924199368,0.117787965463446,0.554148808853529));
#17585=DIRECTION('center_axis',(1.,-9.78147600733805E-16,2.0791169081776E-16));
#17586=DIRECTION('ref_axis',(4.19950331238945E-31,-0.20791169081776,-0.978147600733806));
#17587=DIRECTION('center_axis',(0.,-0.20791169081776,-0.978147600733805));
#17588=DIRECTION('ref_axis',(-1.04747777942724E-15,-0.978147600733805,0.20791169081776));
#17589=DIRECTION('center_axis',(-1.,9.78147600733805E-16,-2.0791169081776E-16));
#17590=DIRECTION('ref_axis',(-7.79618225341413E-32,0.20791169081776,0.978147600733805));
#17591=DIRECTION('center_axis',(0.566528822887065,-0.171327949765012,-0.80603463105968));
#17592=DIRECTION('ref_axis',(-0.824041924199368,-0.117787965463444,-0.55414880885353));
#17593=DIRECTION('center_axis',(-0.824041924199368,0.117787965463446,0.554148808853529));
#17594=DIRECTION('ref_axis',(0.566528822887065,0.17132794976501,0.80603463105968));
#17595=DIRECTION('center_axis',(0.,-0.20791169081776,-0.978147600733805));
#17596=DIRECTION('ref_axis',(-1.01403901935241E-15,-0.978147600733806,0.20791169081776));
#17597=DIRECTION('center_axis',(1.,0.,0.));
#17598=DIRECTION('ref_axis',(0.,0.20791169081776,0.978147600733805));
#17599=DIRECTION('center_axis',(-1.,5.98922883417366E-17,-1.27304988804691E-17));
#17600=DIRECTION('ref_axis',(6.12303176911189E-17,0.978147600733805,-0.20791169081776));
#17601=DIRECTION('',(-1.,0.,0.));
#17602=DIRECTION('center_axis',(-1.,0.,0.));
#17603=DIRECTION('ref_axis',(0.,-0.20791169081776,-0.978147600733805));
#17604=DIRECTION('',(-1.,0.,0.));
#17605=DIRECTION('',(-1.,0.,0.));
#17606=DIRECTION('',(-1.,0.,0.));
#17607=DIRECTION('center_axis',(-1.,0.,0.));
#17608=DIRECTION('ref_axis',(0.,-0.20791169081776,-0.978147600733805));
#17609=DIRECTION('',(-1.,0.,0.));
#17610=DIRECTION('center_axis',(-1.,5.98922883417366E-17,-1.27304988804691E-17));
#17611=DIRECTION('ref_axis',(6.12303176911189E-17,0.978147600733805,-0.20791169081776));
#17612=DIRECTION('center_axis',(-1.,0.,0.));
#17613=DIRECTION('ref_axis',(0.,-0.20791169081776,-0.978147600733805));
#17614=DIRECTION('',(-1.,0.,0.));
#17615=DIRECTION('',(-1.,0.,0.));
#17616=DIRECTION('',(-1.,0.,0.));
#17617=DIRECTION('center_axis',(-1.,0.,0.));
#17618=DIRECTION('ref_axis',(0.,-0.20791169081776,-0.978147600733805));
#17619=DIRECTION('center_axis',(-1.,0.,0.));
#17620=DIRECTION('ref_axis',(0.,-0.20791169081776,-0.978147600733805));
#17621=DIRECTION('',(-1.,0.,0.));
#17622=DIRECTION('',(-1.,0.,0.));
#17623=DIRECTION('',(-1.,0.,0.));
#17624=DIRECTION('center_axis',(-1.,0.,0.));
#17625=DIRECTION('ref_axis',(0.,-0.20791169081776,-0.978147600733805));
#17626=DIRECTION('',(-1.,0.,0.));
#17627=DIRECTION('',(-1.,0.,0.));
#17628=DIRECTION('',(-1.,0.,0.));
#17629=DIRECTION('center_axis',(-1.,0.,0.));
#17630=DIRECTION('ref_axis',(0.,0.20791169081776,0.978147600733805));
#17631=DIRECTION('',(-1.,0.,0.));
#17632=DIRECTION('center_axis',(-1.,0.,0.));
#17633=DIRECTION('ref_axis',(0.,0.20791169081776,0.978147600733805));
#17634=DIRECTION('',(-1.,0.,0.));
#17635=DIRECTION('center_axis',(-1.,0.,0.));
#17636=DIRECTION('ref_axis',(0.,-0.20791169081776,-0.978147600733805));
#17637=DIRECTION('',(-1.,0.,0.));
#17638=DIRECTION('',(-1.,0.,0.));
#17639=DIRECTION('',(-1.,0.,0.));
#17640=DIRECTION('',(-1.,0.,0.));
#17641=DIRECTION('',(-1.,0.,0.));
#17642=DIRECTION('center_axis',(-1.,0.,0.));
#17643=DIRECTION('ref_axis',(0.,-0.20791169081776,-0.978147600733805));
#17644=DIRECTION('',(-1.,0.,0.));
#17645=DIRECTION('',(-1.,0.,0.));
#17646=DIRECTION('',(-1.,0.,0.));
#17647=DIRECTION('',(-1.,0.,0.));
#17648=DIRECTION('',(-1.,0.,0.));
#17649=DIRECTION('center_axis',(-1.48029736616688E-16,-0.20791169081776,
-0.978147600733806));
#17650=DIRECTION('ref_axis',(-1.,1.1842378929335E-15,-2.08166817117217E-16));
#17651=DIRECTION('center_axis',(-1.E-15,-0.978147600733805,0.20791169081776));
#17652=DIRECTION('ref_axis',(2.00292312395533E-31,0.20791169081776,0.978147600733806));
#17653=DIRECTION('center_axis',(-1.,9.78147600733805E-16,-2.0791169081776E-16));
#17654=DIRECTION('ref_axis',(-3.70646524662632E-31,0.20791169081776,0.978147600733806));
#17655=DIRECTION('center_axis',(0.,0.20791169081776,0.978147600733805));
#17656=DIRECTION('ref_axis',(1.01403901935241E-15,0.978147600733806,-0.20791169081776));
#17657=DIRECTION('center_axis',(-0.824041924199368,-0.117787965463444,-0.55414880885353));
#17658=DIRECTION('ref_axis',(-0.566528822887065,0.171327949765011,0.80603463105968));
#17659=DIRECTION('center_axis',(0.566528822887065,0.171327949765011,0.80603463105968));
#17660=DIRECTION('ref_axis',(0.824041924199368,-0.117787965463446,-0.554148808853529));
#17661=DIRECTION('center_axis',(-1.,9.78147600733805E-16,-2.0791169081776E-16));
#17662=DIRECTION('ref_axis',(-7.79618225341413E-32,0.20791169081776,0.978147600733805));
#17663=DIRECTION('center_axis',(0.,0.20791169081776,0.978147600733805));
#17664=DIRECTION('ref_axis',(1.04747777942724E-15,0.978147600733805,-0.20791169081776));
#17665=DIRECTION('center_axis',(1.,-9.78147600733805E-16,2.0791169081776E-16));
#17666=DIRECTION('ref_axis',(4.19950331238945E-31,-0.20791169081776,-0.978147600733806));
#17667=DIRECTION('center_axis',(-0.566528822887065,0.171327949765012,0.80603463105968));
#17668=DIRECTION('ref_axis',(0.824041924199368,0.117787965463444,0.55414880885353));
#17669=DIRECTION('center_axis',(0.824041924199368,-0.117787965463446,-0.554148808853529));
#17670=DIRECTION('ref_axis',(-0.566528822887065,-0.17132794976501,-0.80603463105968));
#17671=DIRECTION('center_axis',(0.,0.20791169081776,0.978147600733805));
#17672=DIRECTION('ref_axis',(1.01403901935241E-15,0.978147600733806,-0.20791169081776));
#17673=DIRECTION('center_axis',(1.,-9.78147600733805E-16,2.0791169081776E-16));
#17674=DIRECTION('ref_axis',(2.21166036268998E-31,-0.20791169081776,-0.978147600733805));
#17675=DIRECTION('center_axis',(0.,-0.20791169081776,-0.978147600733805));
#17676=DIRECTION('ref_axis',(-1.01403901935241E-15,-0.978147600733806,0.20791169081776));
#17677=DIRECTION('center_axis',(0.824041924199368,0.117787965463444,0.55414880885353));
#17678=DIRECTION('ref_axis',(0.566528822887065,-0.171327949765011,-0.80603463105968));
#17679=DIRECTION('center_axis',(-0.566528822887065,-0.171327949765011,-0.80603463105968));
#17680=DIRECTION('ref_axis',(-0.824041924199368,0.117787965463446,0.554148808853529));
#17681=DIRECTION('center_axis',(1.,-9.78147600733805E-16,2.0791169081776E-16));
#17682=DIRECTION('ref_axis',(4.19950331238945E-31,-0.20791169081776,-0.978147600733806));
#17683=DIRECTION('center_axis',(0.,-0.20791169081776,-0.978147600733805));
#17684=DIRECTION('ref_axis',(-1.04747777942724E-15,-0.978147600733805,0.20791169081776));
#17685=DIRECTION('center_axis',(-1.,9.78147600733805E-16,-2.0791169081776E-16));
#17686=DIRECTION('ref_axis',(-7.79618225341413E-32,0.20791169081776,0.978147600733805));
#17687=DIRECTION('center_axis',(0.566528822887065,-0.171327949765012,-0.80603463105968));
#17688=DIRECTION('ref_axis',(-0.824041924199368,-0.117787965463444,-0.55414880885353));
#17689=DIRECTION('center_axis',(-0.824041924199368,0.117787965463446,0.554148808853529));
#17690=DIRECTION('ref_axis',(0.566528822887065,0.17132794976501,0.80603463105968));
#17691=DIRECTION('center_axis',(0.,-0.20791169081776,-0.978147600733805));
#17692=DIRECTION('ref_axis',(-1.01403901935241E-15,-0.978147600733806,0.20791169081776));
#17693=DIRECTION('center_axis',(1.E-15,0.978147600733805,-0.20791169081776));
#17694=DIRECTION('ref_axis',(2.24944215683689E-31,0.20791169081776,0.978147600733806));
#17695=DIRECTION('center_axis',(-1.E-15,-0.978147600733805,0.20791169081776));
#17696=DIRECTION('ref_axis',(2.00292312395533E-31,0.20791169081776,0.978147600733806));
#17697=DIRECTION('center_axis',(-1.E-15,-0.978147600733805,0.20791169081776));
#17698=DIRECTION('ref_axis',(2.00292312395533E-31,0.20791169081776,0.978147600733806));
#17699=DIRECTION('center_axis',(-1.E-15,-0.978147600733805,0.20791169081776));
#17700=DIRECTION('ref_axis',(2.00292312395533E-31,0.20791169081776,0.978147600733806));
#17701=DIRECTION('',(-1.E-15,-0.978147600733806,0.20791169081776));
#17702=DIRECTION('center_axis',(-1.E-15,-0.978147600733805,0.20791169081776));
#17703=DIRECTION('ref_axis',(2.00292312395533E-31,0.20791169081776,0.978147600733806));
#17704=DIRECTION('center_axis',(-1.E-15,-0.978147600733805,0.20791169081776));
#17705=DIRECTION('ref_axis',(2.00292312395533E-31,0.20791169081776,0.978147600733806));
#17706=DIRECTION('center_axis',(0.,-0.978147600733806,0.20791169081776));
#17707=DIRECTION('ref_axis',(0.,-0.20791169081776,-0.978147600733805));
#17708=DIRECTION('center_axis',(-4.56588875816933E-15,0.978147600733806,
-0.207911690817759));
#17709=DIRECTION('ref_axis',(-4.8480728466622E-14,0.207911690817759,0.978147600733806));
#17710=DIRECTION('',(-7.52746977976284E-33,0.20791169081776,0.978147600733805));
#17711=DIRECTION('center_axis',(0.,-0.978147600733806,0.20791169081776));
#17712=DIRECTION('ref_axis',(0.,-0.20791169081776,-0.978147600733805));
#17713=DIRECTION('',(-7.52746977976284E-33,0.20791169081776,0.978147600733805));
#17714=DIRECTION('center_axis',(0.,0.978147600733806,-0.20791169081776));
#17715=DIRECTION('ref_axis',(0.,0.20791169081776,0.978147600733805));
#17716=DIRECTION('center_axis',(1.28919211995368E-14,0.978147600733805,
-0.20791169081776));
#17717=DIRECTION('ref_axis',(-1.52730138049065E-13,0.20791169081776,0.978147600733805));
#17718=DIRECTION('',(-7.52746977976284E-33,-0.20791169081776,-0.978147600733805));
#17719=DIRECTION('center_axis',(1.E-15,0.978147600733805,-0.20791169081776));
#17720=DIRECTION('ref_axis',(-1.,9.78147600733805E-16,-2.0791169081776E-16));
#17721=DIRECTION('center_axis',(-0.824041924199368,-0.117787965463444,-0.55414880885353));
#17722=DIRECTION('ref_axis',(-9.98343400872365E-16,-0.978147600733805,0.20791169081776));
#17723=DIRECTION('',(-1.E-15,-0.978147600733805,0.20791169081776));
#17724=DIRECTION('',(-0.566528822887065,0.171327949765012,0.80603463105968));
#17725=DIRECTION('',(1.E-15,0.978147600733805,-0.20791169081776));
#17726=DIRECTION('center_axis',(0.566528822887065,0.171327949765011,0.80603463105968));
#17727=DIRECTION('ref_axis',(-9.8574048948753E-16,-0.978147600733805,0.20791169081776));
#17728=DIRECTION('',(0.824041924199368,-0.117787965463446,-0.554148808853529));
#17729=DIRECTION('',(1.E-15,0.978147600733805,-0.20791169081776));
#17730=DIRECTION('center_axis',(1.06123031769112E-15,0.978147600733805,
-0.20791169081776));
#17731=DIRECTION('ref_axis',(1.,-1.03803988907554E-15,2.20642189698229E-16));
#17732=DIRECTION('',(1.,-1.03803988907554E-15,2.20642189698229E-16));
#17733=DIRECTION('',(0.,0.20791169081776,0.978147600733805));
#17734=DIRECTION('',(-1.,1.03803988907554E-15,-2.20642189698229E-16));
#17735=DIRECTION('',(0.566528822887065,0.17132794976501,0.80603463105968));
#17736=DIRECTION('',(-0.824041924199368,-0.117787965463444,-0.55414880885353));
#17737=DIRECTION('',(0.,0.20791169081776,0.978147600733805));
#17738=DIRECTION('',(-1.,1.03803988907554E-15,-2.20642189698229E-16));
#17739=DIRECTION('',(0.,-0.20791169081776,-0.978147600733805));
#17740=DIRECTION('',(-0.824041924199368,0.117787965463446,0.554148808853529));
#17741=DIRECTION('',(0.566528822887065,-0.171327949765012,-0.80603463105968));
#17742=DIRECTION('',(-1.,1.03803988907554E-15,-2.20642189698229E-16));
#17743=DIRECTION('',(0.,-0.20791169081776,-0.978147600733805));
#17744=DIRECTION('',(1.,-1.03803988907554E-15,2.20642189698229E-16));
#17745=DIRECTION('',(-0.566528822887065,-0.17132794976501,-0.80603463105968));
#17746=DIRECTION('',(0.824041924199368,0.117787965463444,0.55414880885353));
#17747=DIRECTION('',(0.,-0.20791169081776,-0.978147600733805));
#17748=DIRECTION('',(1.,-1.03803988907554E-15,2.20642189698229E-16));
#17749=DIRECTION('',(0.,0.20791169081776,0.978147600733805));
#17750=DIRECTION('center_axis',(-2.46519032881566E-32,0.20791169081776,
0.978147600733805));
#17751=DIRECTION('ref_axis',(1.E-15,0.978147600733805,-0.20791169081776));
#17752=DIRECTION('',(1.E-15,0.978147600733805,-0.20791169081776));
#17753=DIRECTION('',(1.E-15,0.978147600733805,-0.20791169081776));
#17754=DIRECTION('center_axis',(1.,-9.78147600733805E-16,2.0791169081776E-16));
#17755=DIRECTION('ref_axis',(2.70889472931338E-32,-0.20791169081776,-0.978147600733805));
#17756=DIRECTION('',(-1.E-15,-0.978147600733805,0.20791169081776));
#17757=DIRECTION('center_axis',(-0.566528822887065,0.171327949765012,0.80603463105968));
#17758=DIRECTION('ref_axis',(1.0068127165452E-15,0.978147600733805,-0.20791169081776));
#17759=DIRECTION('',(1.E-15,0.978147600733805,-0.20791169081776));
#17760=DIRECTION('center_axis',(0.824041924199368,-0.117787965463446,-0.554148808853529));
#17761=DIRECTION('ref_axis',(-0.566528822887065,-0.171327949765011,-0.80603463105968));
#17762=DIRECTION('',(1.E-15,0.978147600733805,-0.20791169081776));
#17763=DIRECTION('center_axis',(-2.46519032881566E-32,0.20791169081776,
0.978147600733805));
#17764=DIRECTION('ref_axis',(1.E-15,0.978147600733805,-0.20791169081776));
#17765=DIRECTION('',(1.E-15,0.978147600733805,-0.20791169081776));
#17766=DIRECTION('center_axis',(1.,-9.78147600733805E-16,2.0791169081776E-16));
#17767=DIRECTION('ref_axis',(2.70889472931338E-32,-0.20791169081776,-0.978147600733805));
#17768=DIRECTION('',(1.E-15,0.978147600733805,-0.20791169081776));
#17769=DIRECTION('center_axis',(2.46519032881566E-32,-0.20791169081776,
-0.978147600733805));
#17770=DIRECTION('ref_axis',(1.,-9.78147600733805E-16,2.0791169081776E-16));
#17771=DIRECTION('',(-1.E-15,-0.978147600733805,0.20791169081776));
#17772=DIRECTION('center_axis',(0.824041924199368,0.117787965463444,0.55414880885353));
#17773=DIRECTION('ref_axis',(-9.98343400872365E-16,-0.978147600733805,0.20791169081776));
#17774=DIRECTION('',(1.E-15,0.978147600733805,-0.20791169081776));
#17775=DIRECTION('center_axis',(-0.566528822887065,-0.171327949765011,-0.80603463105968));
#17776=DIRECTION('ref_axis',(-9.8574048948753E-16,-0.978147600733805,0.20791169081776));
#17777=DIRECTION('',(1.E-15,0.978147600733805,-0.20791169081776));
#17778=DIRECTION('center_axis',(1.,-9.78147600733805E-16,2.0791169081776E-16));
#17779=DIRECTION('ref_axis',(2.70889472931338E-32,-0.20791169081776,-0.978147600733805));
#17780=DIRECTION('',(1.E-15,0.978147600733805,-0.20791169081776));
#17781=DIRECTION('center_axis',(2.46519032881566E-32,-0.20791169081776,
-0.978147600733805));
#17782=DIRECTION('ref_axis',(1.,-9.78147600733805E-16,2.0791169081776E-16));
#17783=DIRECTION('',(1.E-15,0.978147600733805,-0.20791169081776));
#17784=DIRECTION('center_axis',(-1.,9.78147600733805E-16,-2.0791169081776E-16));
#17785=DIRECTION('ref_axis',(1.E-15,0.978147600733805,-0.20791169081776));
#17786=DIRECTION('',(-1.E-15,-0.978147600733805,0.20791169081776));
#17787=DIRECTION('center_axis',(0.566528822887065,-0.171327949765012,-0.80603463105968));
#17788=DIRECTION('ref_axis',(0.824041924199368,0.117787965463444,0.55414880885353));
#17789=DIRECTION('',(1.E-15,0.978147600733805,-0.20791169081776));
#17790=DIRECTION('center_axis',(-0.824041924199368,0.117787965463446,0.554148808853529));
#17791=DIRECTION('ref_axis',(1.00985717000555E-15,0.978147600733805,-0.20791169081776));
#17792=DIRECTION('',(1.E-15,0.978147600733805,-0.20791169081776));
#17793=DIRECTION('center_axis',(2.46519032881566E-32,-0.20791169081776,
-0.978147600733805));
#17794=DIRECTION('ref_axis',(1.,-9.78147600733805E-16,2.0791169081776E-16));
#17795=DIRECTION('',(1.E-15,0.978147600733805,-0.20791169081776));
#17796=DIRECTION('center_axis',(-1.,9.78147600733805E-16,-2.0791169081776E-16));
#17797=DIRECTION('ref_axis',(1.E-15,0.978147600733805,-0.20791169081776));
#17798=DIRECTION('',(1.E-15,0.978147600733805,-0.20791169081776));
#17799=DIRECTION('center_axis',(-2.46519032881566E-32,0.20791169081776,
0.978147600733805));
#17800=DIRECTION('ref_axis',(1.E-15,0.978147600733805,-0.20791169081776));
#17801=DIRECTION('center_axis',(-1.,9.78147600733805E-16,-2.0791169081776E-16));
#17802=DIRECTION('ref_axis',(1.E-15,0.978147600733805,-0.20791169081776));
#17803=DIRECTION('center_axis',(1.E-15,0.978147600733805,-0.20791169081776));
#17804=DIRECTION('ref_axis',(-1.,9.78147600733805E-16,-2.0791169081776E-16));
#17805=DIRECTION('center_axis',(0.,0.978147600733805,-0.20791169081776));
#17806=DIRECTION('ref_axis',(1.,0.,0.));
#17807=DIRECTION('',(0.,-0.20791169081776,-0.978147600733805));
#17808=DIRECTION('center_axis',(0.,0.978147600733805,-0.20791169081776));
#17809=DIRECTION('ref_axis',(1.,0.,0.));
#17810=DIRECTION('center_axis',(-1.,5.98922883417366E-17,-1.27304988804691E-17));
#17811=DIRECTION('ref_axis',(-1.59425458228076E-33,0.20791169081776,0.978147600733805));
#17812=DIRECTION('center_axis',(1.,0.,0.));
#17813=DIRECTION('ref_axis',(0.,0.978147600733805,-0.20791169081776));
#17814=DIRECTION('',(-7.52746977976284E-33,-0.20791169081776,-0.978147600733805));
#17815=DIRECTION('center_axis',(1.,0.,0.));
#17816=DIRECTION('ref_axis',(0.,0.978147600733805,-0.20791169081776));
#17817=DIRECTION('center_axis',(-1.,5.98922883417366E-17,-1.27304988804691E-17));
#17818=DIRECTION('ref_axis',(-1.59425458228076E-33,0.20791169081776,0.978147600733805));
#17819=DIRECTION('center_axis',(0.,0.978147600733805,-0.20791169081776));
#17820=DIRECTION('ref_axis',(1.,0.,0.));
#17821=DIRECTION('',(0.,-0.20791169081776,-0.978147600733805));
#17822=DIRECTION('center_axis',(1.,0.,0.));
#17823=DIRECTION('ref_axis',(0.,0.978147600733805,-0.20791169081776));
#17824=DIRECTION('center_axis',(1.,0.,0.));
#17825=DIRECTION('ref_axis',(0.,0.978147600733805,-0.20791169081776));
#17826=DIRECTION('center_axis',(1.,0.,0.));
#17827=DIRECTION('ref_axis',(0.,-0.978147600733805,0.20791169081776));
#17828=DIRECTION('',(0.,0.20791169081776,0.978147600733805));
#17829=DIRECTION('center_axis',(0.,-0.978147600733805,0.20791169081776));
#17830=DIRECTION('ref_axis',(1.,0.,0.));
#17831=DIRECTION('',(0.,0.20791169081776,0.978147600733805));
#17832=DIRECTION('center_axis',(1.,0.,0.));
#17833=DIRECTION('ref_axis',(0.,-0.978147600733805,0.20791169081776));
#17834=DIRECTION('center_axis',(0.,0.978147600733806,-0.20791169081776));
#17835=DIRECTION('ref_axis',(0.,0.20791169081776,0.978147600733805));
#17836=DIRECTION('center_axis',(1.06123031769112E-15,0.978147600733805,
-0.20791169081776));
#17837=DIRECTION('ref_axis',(1.,-1.03803988907554E-15,2.20642189698229E-16));
#17838=DIRECTION('',(-0.566528822887065,0.171327949765012,0.80603463105968));
#17839=DIRECTION('',(1.,-1.03803988907554E-15,2.20642189698229E-16));
#17840=DIRECTION('',(0.,0.20791169081776,0.978147600733805));
#17841=DIRECTION('',(-1.,1.03803988907554E-15,-2.20642189698229E-16));
#17842=DIRECTION('',(0.566528822887065,0.17132794976501,0.80603463105968));
#17843=DIRECTION('',(-0.824041924199368,-0.117787965463444,-0.55414880885353));
#17844=DIRECTION('',(0.,0.20791169081776,0.978147600733805));
#17845=DIRECTION('',(-1.,1.03803988907554E-15,-2.20642189698229E-16));
#17846=DIRECTION('',(0.,-0.20791169081776,-0.978147600733805));
#17847=DIRECTION('',(-0.824041924199368,0.117787965463446,0.554148808853529));
#17848=DIRECTION('',(0.566528822887065,-0.171327949765012,-0.80603463105968));
#17849=DIRECTION('',(-1.,1.03803988907554E-15,-2.20642189698229E-16));
#17850=DIRECTION('',(0.,-0.20791169081776,-0.978147600733805));
#17851=DIRECTION('',(1.,-1.03803988907554E-15,2.20642189698229E-16));
#17852=DIRECTION('',(-0.566528822887065,-0.17132794976501,-0.80603463105968));
#17853=DIRECTION('',(0.824041924199368,0.117787965463444,0.55414880885353));
#17854=DIRECTION('',(0.,-0.20791169081776,-0.978147600733805));
#17855=DIRECTION('',(1.,-1.03803988907554E-15,2.20642189698229E-16));
#17856=DIRECTION('',(0.,0.20791169081776,0.978147600733805));
#17857=DIRECTION('',(0.824041924199368,-0.117787965463446,-0.554148808853529));
#17858=DIRECTION('center_axis',(-1.,9.78147600733805E-16,-2.0791169081776E-16));
#17859=DIRECTION('ref_axis',(1.E-15,0.978147600733805,-0.20791169081776));
#17860=DIRECTION('',(1.E-15,0.978147600733805,-0.20791169081776));
#17861=DIRECTION('',(1.E-15,0.978147600733805,-0.20791169081776));
#17862=DIRECTION('center_axis',(2.46519032881566E-32,-0.20791169081776,
-0.978147600733805));
#17863=DIRECTION('ref_axis',(1.,-9.78147600733805E-16,2.0791169081776E-16));
#17864=DIRECTION('',(1.E-15,0.978147600733805,-0.20791169081776));
#17865=DIRECTION('center_axis',(-0.824041924199368,0.117787965463446,0.554148808853529));
#17866=DIRECTION('ref_axis',(1.00985717000555E-15,0.978147600733805,-0.20791169081776));
#17867=DIRECTION('',(1.E-15,0.978147600733805,-0.20791169081776));
#17868=DIRECTION('center_axis',(0.566528822887065,-0.171327949765012,-0.80603463105968));
#17869=DIRECTION('ref_axis',(0.824041924199368,0.117787965463444,0.55414880885353));
#17870=DIRECTION('',(-1.E-15,-0.978147600733805,0.20791169081776));
#17871=DIRECTION('center_axis',(-1.,9.78147600733805E-16,-2.0791169081776E-16));
#17872=DIRECTION('ref_axis',(1.E-15,0.978147600733805,-0.20791169081776));
#17873=DIRECTION('',(1.E-15,0.978147600733805,-0.20791169081776));
#17874=DIRECTION('center_axis',(2.46519032881566E-32,-0.20791169081776,
-0.978147600733805));
#17875=DIRECTION('ref_axis',(1.,-9.78147600733805E-16,2.0791169081776E-16));
#17876=DIRECTION('',(1.E-15,0.978147600733805,-0.20791169081776));
#17877=DIRECTION('center_axis',(1.,-9.78147600733805E-16,2.0791169081776E-16));
#17878=DIRECTION('ref_axis',(2.70889472931338E-32,-0.20791169081776,-0.978147600733805));
#17879=DIRECTION('',(1.E-15,0.978147600733805,-0.20791169081776));
#17880=DIRECTION('center_axis',(-0.566528822887065,-0.171327949765011,-0.80603463105968));
#17881=DIRECTION('ref_axis',(-9.8574048948753E-16,-0.978147600733805,0.20791169081776));
#17882=DIRECTION('',(1.E-15,0.978147600733805,-0.20791169081776));
#17883=DIRECTION('center_axis',(0.824041924199368,0.117787965463444,0.55414880885353));
#17884=DIRECTION('ref_axis',(-9.98343400872365E-16,-0.978147600733805,0.20791169081776));
#17885=DIRECTION('',(-1.E-15,-0.978147600733805,0.20791169081776));
#17886=DIRECTION('center_axis',(2.46519032881566E-32,-0.20791169081776,
-0.978147600733805));
#17887=DIRECTION('ref_axis',(1.,-9.78147600733805E-16,2.0791169081776E-16));
#17888=DIRECTION('',(1.E-15,0.978147600733805,-0.20791169081776));
#17889=DIRECTION('center_axis',(1.,-9.78147600733805E-16,2.0791169081776E-16));
#17890=DIRECTION('ref_axis',(2.70889472931338E-32,-0.20791169081776,-0.978147600733805));
#17891=DIRECTION('',(1.E-15,0.978147600733805,-0.20791169081776));
#17892=DIRECTION('center_axis',(-2.46519032881566E-32,0.20791169081776,
0.978147600733805));
#17893=DIRECTION('ref_axis',(1.E-15,0.978147600733805,-0.20791169081776));
#17894=DIRECTION('',(1.E-15,0.978147600733805,-0.20791169081776));
#17895=DIRECTION('center_axis',(0.824041924199368,-0.117787965463446,-0.554148808853529));
#17896=DIRECTION('ref_axis',(-0.566528822887065,-0.171327949765011,-0.80603463105968));
#17897=DIRECTION('',(1.E-15,0.978147600733805,-0.20791169081776));
#17898=DIRECTION('center_axis',(-0.566528822887065,0.171327949765012,0.80603463105968));
#17899=DIRECTION('ref_axis',(1.0068127165452E-15,0.978147600733805,-0.20791169081776));
#17900=DIRECTION('',(-1.E-15,-0.978147600733805,0.20791169081776));
#17901=DIRECTION('center_axis',(1.,-9.78147600733805E-16,2.0791169081776E-16));
#17902=DIRECTION('ref_axis',(2.70889472931338E-32,-0.20791169081776,-0.978147600733805));
#17903=DIRECTION('',(1.E-15,0.978147600733805,-0.20791169081776));
#17904=DIRECTION('center_axis',(-2.46519032881566E-32,0.20791169081776,
0.978147600733805));
#17905=DIRECTION('ref_axis',(1.E-15,0.978147600733805,-0.20791169081776));
#17906=DIRECTION('',(1.E-15,0.978147600733805,-0.20791169081776));
#17907=DIRECTION('center_axis',(-1.,9.78147600733805E-16,-2.0791169081776E-16));
#17908=DIRECTION('ref_axis',(1.E-15,0.978147600733805,-0.20791169081776));
#17909=DIRECTION('',(1.E-15,0.978147600733805,-0.20791169081776));
#17910=DIRECTION('center_axis',(0.566528822887065,0.171327949765011,0.80603463105968));
#17911=DIRECTION('ref_axis',(-9.8574048948753E-16,-0.978147600733805,0.20791169081776));
#17912=DIRECTION('',(1.E-15,0.978147600733805,-0.20791169081776));
#17913=DIRECTION('center_axis',(-0.824041924199368,-0.117787965463444,-0.55414880885353));
#17914=DIRECTION('ref_axis',(-9.98343400872365E-16,-0.978147600733805,0.20791169081776));
#17915=DIRECTION('',(-1.E-15,-0.978147600733805,0.20791169081776));
#17916=DIRECTION('center_axis',(-2.46519032881566E-32,0.20791169081776,
0.978147600733805));
#17917=DIRECTION('ref_axis',(1.E-15,0.978147600733805,-0.20791169081776));
#17918=DIRECTION('center_axis',(1.E-15,0.978147600733805,-0.20791169081776));
#17919=DIRECTION('ref_axis',(-1.,9.78147600733805E-16,-2.0791169081776E-16));
#17920=DIRECTION('center_axis',(1.E-15,0.978147600733805,-0.20791169081776));
#17921=DIRECTION('ref_axis',(-1.,9.78147600733805E-16,-2.0791169081776E-16));
#17922=DIRECTION('center_axis',(0.,0.978147600733805,-0.20791169081776));
#17923=DIRECTION('ref_axis',(1.,0.,0.));
#17924=DIRECTION('center_axis',(5.03209005654235E-16,0.978147600733805,
-0.207911690817761));
#17925=DIRECTION('ref_axis',(-4.65508415806216E-13,0.207911690817761,0.978147600733805));
#17926=DIRECTION('center_axis',(0.,0.978147600733805,-0.20791169081776));
#17927=DIRECTION('ref_axis',(1.,0.,0.));
#17928=DIRECTION('center_axis',(-4.57462732412941E-16,0.978147600733806,
-0.207911690817759));
#17929=DIRECTION('ref_axis',(-2.42086334163375E-13,0.207911690817759,0.978147600733806));
#17930=DIRECTION('center_axis',(0.,0.978147600733805,-0.20791169081776));
#17931=DIRECTION('ref_axis',(1.,0.,0.));
#17932=DIRECTION('center_axis',(-2.49317189165052E-15,0.978147600733805,
-0.207911690817763));
#17933=DIRECTION('ref_axis',(1.26498082100614E-13,0.207911690817763,0.978147600733805));
#17934=DIRECTION('center_axis',(7.77686645101999E-16,0.978147600733806,
-0.207911690817759));
#17935=DIRECTION('ref_axis',(1.70927684112078E-13,0.207911690817759,0.978147600733806));
#17936=DIRECTION('center_axis',(0.,0.978147600733805,-0.20791169081776));
#17937=DIRECTION('ref_axis',(1.,0.,0.));
#34069=CARTESIAN_POINT('',(0.,0.,0.));
#34070=CARTESIAN_POINT('Ctrl Pts',(-1.77573785876366E-15,38.6077491572282,
14.5682581662533));
#34071=CARTESIAN_POINT('Ctrl Pts',(-1.77573785876366E-15,37.4339720363476,
14.8177521952346));
#34072=CARTESIAN_POINT('Ctrl Pts',(29.,38.6077491572282,14.5682581662533));
#34073=CARTESIAN_POINT('Ctrl Pts',(29.,37.4339720363476,14.8177521952346));
#34074=CARTESIAN_POINT('Ctrl Pts',(29.,32.3703984326954,-14.7761698557608));
#34075=CARTESIAN_POINT('Ctrl Pts',(29.,31.1966213118148,-14.5266758267795));
#34076=CARTESIAN_POINT('Ctrl Pts',(0.,32.3703984326954,-14.7761698557608));
#34077=CARTESIAN_POINT('Ctrl Pts',(0.,31.1966213118148,-14.5266758267795));
#34078=CARTESIAN_POINT('',(-1.77573785876366E-15,38.6077491572282,14.5682581662533));
#34079=CARTESIAN_POINT('',(13.9832936034398,36.3141977378119,3.77794710083046));
#34080=CARTESIAN_POINT('Origin',(6.26496290550477E-13,35.489073794962,-0.103955844753016));
#34081=CARTESIAN_POINT('',(-1.77573785876366E-15,37.6296015564944,14.7761698570711));
#34082=CARTESIAN_POINT('',(-1.77573785876366E-15,38.6077491572282,14.5682581662533));
#34083=CARTESIAN_POINT('',(13.9832936034398,35.3360501370781,3.98585879164823));
#34084=CARTESIAN_POINT('Origin',(-4.06952304038461E-13,34.5109261942279,
0.103955846063604));
#34085=CARTESIAN_POINT('',(13.9832936034398,33.6858022513779,-3.77794709952022));
#34086=CARTESIAN_POINT('Origin',(1.71995750974929E-11,34.510926194228,0.103955846063976));
#34087=CARTESIAN_POINT('',(0.,31.3922508319616,-14.5682581649431));
#34088=CARTESIAN_POINT('Origin',(-7.105427357601E-14,34.510926194228,0.10395584606411));
#34089=CARTESIAN_POINT('',(0.,32.3703984326954,-14.7761698557608));
#34090=CARTESIAN_POINT('',(0.,32.3703984326954,-14.7761698557608));
#34091=CARTESIAN_POINT('',(13.9832936034398,34.6639498521117,-3.98585879033799));
#34092=CARTESIAN_POINT('Origin',(-2.22044604925031E-14,35.4890737949618,
-0.103955844753743));
#34093=CARTESIAN_POINT('Origin',(2.6754154447417E-11,35.4890737949615,-0.103955844754103));
#34094=CARTESIAN_POINT('Origin',(7.49999972068901,37.9344427967963,-0.62373507179816));
#34095=CARTESIAN_POINT('',(8.91421328306212,32.6156398209602,3.21167037016454));
#34096=CARTESIAN_POINT('',(6.08578615831592,32.6156398209602,3.21167037016456));
#34097=CARTESIAN_POINT('Origin',(7.499999720689,32.0655571923935,0.6237350731084));
#34098=CARTESIAN_POINT('',(6.08578615831588,31.5154745638267,-1.96420022394774));
#34099=CARTESIAN_POINT('Origin',(7.499999720689,32.0655571923935,0.6237350731084));
#34100=CARTESIAN_POINT('',(7.499999720689,31.4418221199402,-2.31070772909302));
#34101=CARTESIAN_POINT('Origin',(7.499999720689,32.0655571923935,0.6237350731084));
#34102=CARTESIAN_POINT('',(7.499999720689,29.8805494572643,-1.97884898008522));
#34103=CARTESIAN_POINT('',(7.49999972068901,37.310707724343,-3.55817787399958));
#34104=CARTESIAN_POINT('Origin',(7.499999720689,30.5042845297176,0.955593822116194));
#34105=CARTESIAN_POINT('',(8.91421328306212,31.5154745638267,-1.96420022394774));
#34106=CARTESIAN_POINT('Origin',(7.499999720689,32.0655571923935,0.6237350731084));
#34107=CARTESIAN_POINT('Origin',(7.499999720689,32.0655571923935,0.6237350731084));
#34108=CARTESIAN_POINT('Origin',(7.49999972068907,35.5868885550352,-0.124747013835536));
#34109=CARTESIAN_POINT('',(5.949999720689,29.8493353829967,0.698650580301697));
#34110=CARTESIAN_POINT('',(5.949999720689,30.0104669433805,1.4567149708704));
#34111=CARTESIAN_POINT('Origin',(5.949999720689,35.5868885550352,-0.124747013835536));
#34112=CARTESIAN_POINT('',(6.846093470689,29.8458529108876,1.49170476361971));
#34113=CARTESIAN_POINT('Origin',(7.49999972068907,35.6674543352271,0.254285181448814));
#34114=CARTESIAN_POINT('',(6.259999720689,30.2320748221203,2.28115611924892));
#34115=CARTESIAN_POINT('Origin',(7.23686974721422,35.5492769441233,-0.301695730997491));
#34116=CARTESIAN_POINT('',(7.112499720689,29.9012418847696,1.7522893978777));
#34117=CARTESIAN_POINT('Origin',(7.68090157745298,35.6415963527252,0.13263293839996));
#34118=CARTESIAN_POINT('',(7.112499720689,30.2521642839561,2.59381155672345));
#34119=CARTESIAN_POINT('Origin',(7.112499720689,35.5868885550352,-0.124747013835536));
#34120=CARTESIAN_POINT('',(7.887499720689,30.2521642839561,2.59381155672345));
#34121=CARTESIAN_POINT('Origin',(7.49999972068907,35.9091516758027,1.39138176730186));
#34122=CARTESIAN_POINT('',(7.887499720689,29.9012418847695,1.7522893978777));
#34123=CARTESIAN_POINT('Origin',(7.88749972068901,35.5868885550352,-0.124747013835536));
#34124=CARTESIAN_POINT('',(8.739999720689,30.2320748221202,2.28115611924892));
#34125=CARTESIAN_POINT('Origin',(7.31909786392512,35.6415963527252,0.132632938400021));
#34126=CARTESIAN_POINT('',(8.153905970689,29.8458529108876,1.49170476361971));
#34127=CARTESIAN_POINT('Origin',(7.76312969416383,35.5492769441233,-0.30169573099743));
#34128=CARTESIAN_POINT('',(9.049999720689,30.0104669433804,1.45671497087041));
#34129=CARTESIAN_POINT('Origin',(7.49999972068907,35.6674543352271,0.254285181448814));
#34130=CARTESIAN_POINT('',(9.049999720689,29.8493353829967,0.698650580301706));
#34131=CARTESIAN_POINT('Origin',(9.04999972068901,35.5868885550352,-0.124747013835536));
#34132=CARTESIAN_POINT('',(8.153905970689,29.6847213505039,0.733640373051015));
#34133=CARTESIAN_POINT('Origin',(7.49999972068907,35.5063227748433,-0.503779209119886));
#34134=CARTESIAN_POINT('',(8.739999720689,29.7164538288922,-0.144649930570914));
#34135=CARTESIAN_POINT('Origin',(7.76312969416383,35.624500165947,0.0522017033263585));
#34136=CARTESIAN_POINT('',(7.887499720689,29.6293323766219,0.473055738793025));
#34137=CARTESIAN_POINT('Origin',(7.31909786392512,35.5321807573452,-0.382126966071094));
#34138=CARTESIAN_POINT('',(7.887499720689,29.607638042421,-0.438446005551347));
#34139=CARTESIAN_POINT('Origin',(7.88749972068901,35.5868885550352,-0.124747013835536));
#34140=CARTESIAN_POINT('',(7.112499720689,29.6076380424211,-0.438446005551349));
#34141=CARTESIAN_POINT('Origin',(7.49999972068907,35.2646254342677,-1.64087579497293));
#34142=CARTESIAN_POINT('',(7.112499720689,29.629332376622,0.473055738793022));
#34143=CARTESIAN_POINT('Origin',(7.112499720689,35.5868885550352,-0.124747013835536));
#34144=CARTESIAN_POINT('',(6.259999720689,29.7164538288922,-0.144649930570921));
#34145=CARTESIAN_POINT('Origin',(7.68090157745298,35.5321807573452,-0.382126966071032));
#34146=CARTESIAN_POINT('',(6.846093470689,29.6847213505039,0.733640373051013));
#34147=CARTESIAN_POINT('Origin',(7.23686974721422,35.6245001659471,0.0522017033264189));
#34148=CARTESIAN_POINT('Origin',(7.49999972068907,35.5063227748433,-0.503779209119886));
#34149=CARTESIAN_POINT('Origin',(22.5,34.9999999945949,6.55125051005245E-10));
#34150=CARTESIAN_POINT('',(22.5,34.1683532313239,-3.9125904022801));
#34151=CARTESIAN_POINT('Origin',(22.5,34.9999999945949,6.55125051005245E-10));
#34152=CARTESIAN_POINT('',(14.55,34.1683532313239,-3.9125904022801));
#34153=CARTESIAN_POINT('',(22.5,34.1683532313239,-3.9125904022801));
#34154=CARTESIAN_POINT('',(14.55,34.6639498521117,-3.98585879033799));
#34155=CARTESIAN_POINT('Origin',(14.55,34.9999999945949,6.55125051005245E-10));
#34156=CARTESIAN_POINT('',(14.55,34.6639498521117,-3.98585879033799));
#34157=CARTESIAN_POINT('',(-13.9832936034398,34.6639498521117,-3.98585879033799));
#34158=CARTESIAN_POINT('',(14.55,34.6639498521117,-3.98585879033799));
#34159=CARTESIAN_POINT('',(-14.55,34.6639498521117,-3.98585879033799));
#34160=CARTESIAN_POINT('',(14.55,34.6639498521117,-3.98585879033799));
#34161=CARTESIAN_POINT('',(-14.55,34.1683532313239,-3.9125904022801));
#34162=CARTESIAN_POINT('Origin',(-14.55,34.9999999945949,6.55125051005245E-10));
#34163=CARTESIAN_POINT('',(-22.5,34.1683532313239,-3.9125904022801));
#34164=CARTESIAN_POINT('',(22.5,34.1683532313239,-3.9125904022801));
#34165=CARTESIAN_POINT('Origin',(-22.5,34.9999999945949,6.55125051005245E-10));
#34166=CARTESIAN_POINT('',(-14.55,33.6858022513779,-3.77794709952022));
#34167=CARTESIAN_POINT('Origin',(-14.55,34.9999999945949,6.55125051005245E-10));
#34168=CARTESIAN_POINT('',(-13.9832936034398,33.6858022513779,-3.77794709952022));
#34169=CARTESIAN_POINT('',(14.55,33.6858022513779,-3.77794709952022));
#34170=CARTESIAN_POINT('',(14.55,33.6858022513779,-3.77794709952022));
#34171=CARTESIAN_POINT('',(14.55,33.6858022513779,-3.77794709952022));
#34172=CARTESIAN_POINT('',(14.55,33.6858022513779,-3.77794709952022));
#34173=CARTESIAN_POINT('Origin',(14.55,34.9999999945949,6.55125051005245E-10));
#34174=CARTESIAN_POINT('',(-14.55,35.3360501370781,3.98585879164823));
#34175=CARTESIAN_POINT('',(-14.55,36.3141977378119,3.77794710083046));
#34176=CARTESIAN_POINT('Origin',(-14.55,34.9999999945949,6.55125051005245E-10));
#34177=CARTESIAN_POINT('',(-13.9832936034398,36.3141977378119,3.77794710083047));
#34178=CARTESIAN_POINT('',(14.55,36.3141977378119,3.77794710083046));
#34179=CARTESIAN_POINT('',(14.55,36.3141977378119,3.77794710083046));
#34180=CARTESIAN_POINT('',(14.55,36.3141977378119,3.77794710083046));
#34181=CARTESIAN_POINT('',(14.55,36.3141977378119,3.77794710083046));
#34182=CARTESIAN_POINT('',(14.55,35.3360501370781,3.98585879164823));
#34183=CARTESIAN_POINT('Origin',(14.55,34.9999999945949,6.55125051005245E-10));
#34184=CARTESIAN_POINT('',(14.55,35.3360501370781,3.98585879164823));
#34185=CARTESIAN_POINT('',(-13.9832936034398,35.3360501370781,3.98585879164823));
#34186=CARTESIAN_POINT('',(14.55,35.3360501370781,3.98585879164823));
#34187=CARTESIAN_POINT('',(14.55,35.3360501370781,3.98585879164823));
#34188=CARTESIAN_POINT('',(14.55,38.4845254253631,1.96420022525798));
#34189=CARTESIAN_POINT('',(14.55,37.3843601682296,-3.21167036885432));
#34190=CARTESIAN_POINT('Origin',(14.55,34.9999999945949,6.55114870111609E-10));
#34191=CARTESIAN_POINT('',(-14.55,38.4845254253631,1.96420022525798));
#34192=CARTESIAN_POINT('',(14.55,38.4845254253631,1.96420022525798));
#34193=CARTESIAN_POINT('',(-14.55,37.3843601682296,-3.21167036885432));
#34194=CARTESIAN_POINT('Origin',(-14.55,34.9999999945949,6.55114870111609E-10));
#34195=CARTESIAN_POINT('',(14.55,37.3843601682296,-3.21167036885432));
#34196=CARTESIAN_POINT('',(14.55,31.5154745638267,-1.96420022394774));
#34197=CARTESIAN_POINT('',(14.55,32.6156398209602,3.21167037016456));
#34198=CARTESIAN_POINT('Origin',(14.55,34.9999999945949,6.55125051005245E-10));
#34199=CARTESIAN_POINT('',(14.55,31.5154745638267,-1.96420022394774));
#34200=CARTESIAN_POINT('',(14.55,31.5154745638267,-1.96420022394774));
#34201=CARTESIAN_POINT('',(-6.08578624028789,31.5154745638267,-1.96420022394774));
#34202=CARTESIAN_POINT('',(14.55,31.5154745638267,-1.96420022394774));
#34203=CARTESIAN_POINT('',(-8.91421336503412,31.5154745638267,-1.96420022394774));
#34204=CARTESIAN_POINT('',(14.55,31.5154745638267,-1.96420022394774));
#34205=CARTESIAN_POINT('',(-14.55,31.5154745638267,-1.96420022394774));
#34206=CARTESIAN_POINT('',(14.55,31.5154745638267,-1.96420022394774));
#34207=CARTESIAN_POINT('',(-14.55,32.6156398209602,3.21167037016456));
#34208=CARTESIAN_POINT('Origin',(-14.55,34.9999999945949,6.55125051005245E-10));
#34209=CARTESIAN_POINT('',(-8.91421336503407,32.6156398209602,3.21167037016456));
#34210=CARTESIAN_POINT('',(14.55,32.6156398209602,3.21167037016456));
#34211=CARTESIAN_POINT('',(-6.08578624028785,32.6156398209602,3.21167037016452));
#34212=CARTESIAN_POINT('',(14.55,32.6156398209602,3.21167037016456));
#34213=CARTESIAN_POINT('',(14.55,32.6156398209602,3.21167037016456));
#34214=CARTESIAN_POINT('',(14.55,32.6156398209602,3.21167037016456));
#34215=CARTESIAN_POINT('',(14.55,32.6156398209602,3.21167037016456));
#34216=CARTESIAN_POINT('Origin',(-7.49999980266093,35.5868885550352,-0.124747013835536));
#34217=CARTESIAN_POINT('',(-7.499999802661,29.8805494572643,-1.97884898008522));
#34218=CARTESIAN_POINT('Origin',(-7.499999802661,30.5042845297176,0.955593822116194));
#34219=CARTESIAN_POINT('',(-9.049999802661,29.8493353829967,0.698650580301697));
#34220=CARTESIAN_POINT('',(-9.049999802661,30.0104669433805,1.4567149708704));
#34221=CARTESIAN_POINT('Origin',(-9.049999802661,35.5868885550352,-0.124747013835536));
#34222=CARTESIAN_POINT('',(-8.153906052661,29.8458529108876,1.49170476361971));
#34223=CARTESIAN_POINT('Origin',(-7.49999980266093,35.6674543352271,0.254285181448814));
#34224=CARTESIAN_POINT('',(-8.739999802661,30.2320748221203,2.28115611924892));
#34225=CARTESIAN_POINT('Origin',(-7.76312977613578,35.5492769441233,-0.301695730997491));
#34226=CARTESIAN_POINT('',(-7.887499802661,29.9012418847696,1.7522893978777));
#34227=CARTESIAN_POINT('Origin',(-7.31909794589703,35.6415963527252,0.13263293839996));
#34228=CARTESIAN_POINT('',(-7.887499802661,30.2521642839561,2.59381155672345));
#34229=CARTESIAN_POINT('Origin',(-7.887499802661,35.5868885550352,-0.124747013835536));
#34230=CARTESIAN_POINT('',(-7.112499802661,30.2521642839561,2.59381155672345));
#34231=CARTESIAN_POINT('Origin',(-7.49999980266093,35.9091516758027,1.39138176730186));
#34232=CARTESIAN_POINT('',(-7.112499802661,29.9012418847695,1.7522893978777));
#34233=CARTESIAN_POINT('Origin',(-7.112499802661,35.5868885550352,-0.124747013835536));
#34234=CARTESIAN_POINT('',(-6.259999802661,30.2320748221202,2.28115611924892));
#34235=CARTESIAN_POINT('Origin',(-7.68090165942488,35.6415963527252,0.132632938400021));
#34236=CARTESIAN_POINT('',(-6.846093552661,29.8458529108876,1.49170476361971));
#34237=CARTESIAN_POINT('Origin',(-7.23686982918617,35.5492769441233,-0.30169573099743));
#34238=CARTESIAN_POINT('',(-5.949999802661,30.0104669433804,1.45671497087041));
#34239=CARTESIAN_POINT('Origin',(-7.49999980266093,35.6674543352271,0.254285181448814));
#34240=CARTESIAN_POINT('',(-5.949999802661,29.8493353829967,0.698650580301706));
#34241=CARTESIAN_POINT('Origin',(-5.949999802661,35.5868885550352,-0.124747013835536));
#34242=CARTESIAN_POINT('',(-6.846093552661,29.6847213505039,0.733640373051015));
#34243=CARTESIAN_POINT('Origin',(-7.49999980266093,35.5063227748433,-0.503779209119886));
#34244=CARTESIAN_POINT('',(-6.259999802661,29.7164538288922,-0.144649930570914));
#34245=CARTESIAN_POINT('Origin',(-7.23686982918617,35.624500165947,0.0522017033263585));
#34246=CARTESIAN_POINT('',(-7.112499802661,29.6293323766219,0.473055738793025));
#34247=CARTESIAN_POINT('Origin',(-7.68090165942488,35.5321807573452,-0.382126966071094));
#34248=CARTESIAN_POINT('',(-7.112499802661,29.607638042421,-0.438446005551347));
#34249=CARTESIAN_POINT('Origin',(-7.112499802661,35.5868885550352,-0.124747013835536));
#34250=CARTESIAN_POINT('',(-7.887499802661,29.6076380424211,-0.438446005551349));
#34251=CARTESIAN_POINT('Origin',(-7.49999980266093,35.2646254342677,-1.64087579497293));
#34252=CARTESIAN_POINT('',(-7.887499802661,29.629332376622,0.473055738793022));
#34253=CARTESIAN_POINT('Origin',(-7.887499802661,35.5868885550352,-0.124747013835536));
#34254=CARTESIAN_POINT('',(-8.739999802661,29.7164538288922,-0.144649930570921));
#34255=CARTESIAN_POINT('Origin',(-7.31909794589703,35.5321807573452,-0.382126966071032));
#34256=CARTESIAN_POINT('',(-8.153906052661,29.6847213505039,0.733640373051013));
#34257=CARTESIAN_POINT('Origin',(-7.76312977613578,35.6245001659471,0.0522017033264189));
#34258=CARTESIAN_POINT('Origin',(-7.49999980266093,35.5063227748433,-0.503779209119886));
#34259=CARTESIAN_POINT('Origin',(-7.49999980266099,37.9344427967963,-0.62373507179816));
#34260=CARTESIAN_POINT('Origin',(-7.499999802661,32.0655571923935,0.6237350731084));
#34261=CARTESIAN_POINT('Origin',(-7.499999802661,32.0655571923935,0.6237350731084));
#34262=CARTESIAN_POINT('',(-7.499999802661,31.4418221199402,-2.31070772909302));
#34263=CARTESIAN_POINT('Origin',(-7.499999802661,32.0655571923935,0.6237350731084));
#34264=CARTESIAN_POINT('',(-7.49999980266099,37.310707724343,-3.55817787399958));
#34265=CARTESIAN_POINT('Origin',(-7.499999802661,32.0655571923935,0.6237350731084));
#34266=CARTESIAN_POINT('Origin',(-7.499999802661,32.0655571923935,0.6237350731084));
#34267=CARTESIAN_POINT('Origin',(14.55,35.3360501370781,3.98585879164823));
#34268=CARTESIAN_POINT('Origin',(-1.25033317033285E-11,34.5109261942281,
0.103955846063943));
#34269=CARTESIAN_POINT('',(-14.55,35.3360501370781,3.98585879164823));
#34270=CARTESIAN_POINT('Origin',(14.55,35.3360501370781,3.98585879164823));
#34271=CARTESIAN_POINT('',(14.55,35.3360501370781,3.98585879164823));
#34272=CARTESIAN_POINT('Origin',(14.55,34.6639498521117,-3.98585879033799));
#34273=CARTESIAN_POINT('Origin',(1.28297372725683E-11,35.4890737949616,
-0.103955844753872));
#34274=CARTESIAN_POINT('',(-14.55,34.6639498521117,-3.98585879033799));
#34275=CARTESIAN_POINT('Origin',(-10.499999802661,32.0655571923935,0.6237350731084));
#34276=CARTESIAN_POINT('Origin',(-7.887499802661,28.6001199783652,1.3603364920056));
#34277=CARTESIAN_POINT('',(-8.153906052661,31.0282400003182,1.24038062932732));
#34278=CARTESIAN_POINT('',(-8.15390605266101,28.6806857585571,1.73936868728995));
#34279=CARTESIAN_POINT('',(-8.739999802661,31.2054847167403,2.07425145895289));
#34280=CARTESIAN_POINT('',(-7.887499802661,30.9476742201263,0.861348434042974));
#34281=CARTESIAN_POINT('',(-8.739999802661,28.8579304749792,2.57323951691552));
#34282=CARTESIAN_POINT('Origin',(-8.739999802661,28.8579304749792,2.57323951691552));
#34283=CARTESIAN_POINT('',(-7.887499802661,31.0836289742001,1.50096526358531));
#34284=CARTESIAN_POINT('',(-8.739999802661,31.2054847167403,2.07425145895289));
#34285=CARTESIAN_POINT('',(-7.887499802661,28.736074732439,1.99995332154794));
#34286=CARTESIAN_POINT('Origin',(-7.112499802661,31.2699373408939,2.37747721518037));
#34287=CARTESIAN_POINT('',(-9.049999802661,31.0282400003182,1.24038062932732));
#34288=CARTESIAN_POINT('',(-9.049999802661,31.0282400003182,1.24038062932732));
#34289=CARTESIAN_POINT('',(-9.049999802661,30.8671084399344,0.482316238758624));
#34290=CARTESIAN_POINT('',(-9.049999802661,30.8671084399344,0.482316238758624));
#34291=CARTESIAN_POINT('',(-8.153906052661,30.8671084399344,0.482316238758625));
#34292=CARTESIAN_POINT('',(-7.887499802661,30.8671084399344,0.482316238758625));
#34293=CARTESIAN_POINT('',(-8.739999802661,30.6898637235123,-0.351554590866945));
#34294=CARTESIAN_POINT('',(-8.739999802661,30.6898637235123,-0.351554590866945));
#34295=CARTESIAN_POINT('',(-7.887499802661,30.8117194660525,0.221731604500634));
#34296=CARTESIAN_POINT('',(-7.499999802661,30.8671084399344,0.482316238758625));
#34297=CARTESIAN_POINT('',(-7.887499802661,30.6254110993588,-0.654780347094424));
#34298=CARTESIAN_POINT('',(-7.887499802661,30.6254110993588,-0.654780347094424));
#34299=CARTESIAN_POINT('',(-7.112499802661,30.6254110993588,-0.654780347094424));
#34300=CARTESIAN_POINT('',(-7.112499802661,30.6254110993588,-0.654780347094424));
#34301=CARTESIAN_POINT('',(-7.112499802661,30.8117194660525,0.221731604500634));
#34302=CARTESIAN_POINT('',(-7.112499802661,30.8671084399344,0.482316238758625));
#34303=CARTESIAN_POINT('',(-6.259999802661,30.6898637235123,-0.351554590866944));
#34304=CARTESIAN_POINT('',(-6.259999802661,30.6898637235123,-0.351554590866944));
#34305=CARTESIAN_POINT('',(-6.846093552661,30.8671084399344,0.482316238758625));
#34306=CARTESIAN_POINT('',(-7.112499802661,30.9476742201263,0.861348434042974));
#34307=CARTESIAN_POINT('',(-5.949999802661,30.8671084399344,0.482316238758625));
#34308=CARTESIAN_POINT('',(-5.949999802661,30.8671084399344,0.482316238758625));
#34309=CARTESIAN_POINT('',(-5.949999802661,31.0282400003182,1.24038062932732));
#34310=CARTESIAN_POINT('',(-5.949999802661,31.0282400003182,1.24038062932732));
#34311=CARTESIAN_POINT('',(-6.846093552661,31.0282400003182,1.24038062932732));
#34312=CARTESIAN_POINT('',(-7.112499802661,31.0282400003182,1.24038062932732));
#34313=CARTESIAN_POINT('',(-6.259999802661,31.2054847167403,2.07425145895289));
#34314=CARTESIAN_POINT('',(-6.259999802661,31.2054847167403,2.07425145895289));
#34315=CARTESIAN_POINT('',(-7.112499802661,31.0836289742001,1.50096526358531));
#34316=CARTESIAN_POINT('',(-7.499999802661,31.0282400003182,1.24038062932732));
#34317=CARTESIAN_POINT('',(-7.112499802661,31.2699373408939,2.37747721518037));
#34318=CARTESIAN_POINT('',(-7.112499802661,31.2699373408939,2.37747721518037));
#34319=CARTESIAN_POINT('',(-7.887499802661,31.2699373408939,2.37747721518037));
#34320=CARTESIAN_POINT('',(-7.887499802661,31.2699373408939,2.37747721518037));
#34321=CARTESIAN_POINT('',(-7.887499802661,31.0282400003182,1.24038062932732));
#34322=CARTESIAN_POINT('Origin',(-7.887499802661,28.9223830991327,2.876465273143));
#34323=CARTESIAN_POINT('',(-7.887499802661,28.9223830991327,2.876465273143));
#34324=CARTESIAN_POINT('',(-7.112499802661,28.9223830991327,2.876465273143));
#34325=CARTESIAN_POINT('Origin',(-7.112499802661,28.9223830991327,2.876465273143));
#34326=CARTESIAN_POINT('',(-7.112499802661,28.736074732439,1.99995332154794));
#34327=CARTESIAN_POINT('Origin',(-7.49999980266101,28.6806857585571,1.73936868728995));
#34328=CARTESIAN_POINT('',(-6.259999802661,28.8579304749792,2.57323951691552));
#34329=CARTESIAN_POINT('Origin',(-6.259999802661,28.8579304749792,2.57323951691552));
#34330=CARTESIAN_POINT('',(-6.846093552661,28.6806857585571,1.73936868728995));
#34331=CARTESIAN_POINT('Origin',(-7.112499802661,28.6806857585571,1.73936868728995));
#34332=CARTESIAN_POINT('',(-5.949999802661,28.6806857585571,1.73936868728995));
#34333=CARTESIAN_POINT('Origin',(-5.949999802661,28.6806857585571,1.73936868728995));
#34334=CARTESIAN_POINT('',(-5.949999802661,28.5195541981733,0.981304296721249));
#34335=CARTESIAN_POINT('Origin',(-5.949999802661,28.5195541981733,0.981304296721249));
#34336=CARTESIAN_POINT('',(-6.846093552661,28.5195541981733,0.981304296721249));
#34337=CARTESIAN_POINT('Origin',(-7.112499802661,28.6001199783652,1.3603364920056));
#34338=CARTESIAN_POINT('',(-6.259999802661,28.3423094817512,0.14743346709568));
#34339=CARTESIAN_POINT('Origin',(-6.259999802661,28.3423094817512,0.14743346709568));
#34340=CARTESIAN_POINT('',(-7.112499802661,28.4641652242914,0.720719662463259));
#34341=CARTESIAN_POINT('Origin',(-7.112499802661,28.5195541981733,0.981304296721249));
#34342=CARTESIAN_POINT('',(-7.112499802661,28.2778568575977,-0.1557922891318));
#34343=CARTESIAN_POINT('Origin',(-7.112499802661,28.2778568575977,-0.1557922891318));
#34344=CARTESIAN_POINT('',(-7.887499802661,28.2778568575977,-0.1557922891318));
#34345=CARTESIAN_POINT('Origin',(-7.887499802661,28.2778568575977,-0.1557922891318));
#34346=CARTESIAN_POINT('',(-7.887499802661,28.4641652242914,0.720719662463258));
#34347=CARTESIAN_POINT('Origin',(-7.49999980266101,28.5195541981733,0.981304296721249));
#34348=CARTESIAN_POINT('',(-8.739999802661,28.3423094817512,0.14743346709568));
#34349=CARTESIAN_POINT('Origin',(-8.739999802661,28.3423094817512,0.14743346709568));
#34350=CARTESIAN_POINT('',(-8.15390605266101,28.5195541981733,0.981304296721249));
#34351=CARTESIAN_POINT('Origin',(-7.887499802661,28.5195541981733,0.981304296721249));
#34352=CARTESIAN_POINT('',(-9.049999802661,28.5195541981733,0.981304296721248));
#34353=CARTESIAN_POINT('Origin',(-9.049999802661,28.5195541981733,0.981304296721248));
#34354=CARTESIAN_POINT('',(-9.049999802661,28.6806857585571,1.73936868728995));
#34355=CARTESIAN_POINT('Origin',(-9.049999802661,28.6806857585571,1.73936868728995));
#34356=CARTESIAN_POINT('Origin',(-7.887499802661,28.6806857585571,1.73936868728995));
#34357=CARTESIAN_POINT('Origin',(-10.499999802661,32.0655571923935,0.6237350731084));
#34358=CARTESIAN_POINT('Origin',(14.55,32.6156398209602,3.21167037016456));
#34359=CARTESIAN_POINT('',(-14.55,32.6156398209602,3.21167037016456));
#34360=CARTESIAN_POINT('Origin',(14.55,32.6156398209602,3.21167037016456));
#34361=CARTESIAN_POINT('Origin',(22.5,34.9999999945949,6.55125051005245E-10));
#34362=CARTESIAN_POINT('Origin',(14.55,32.6768994428521,0.493790266347305));
#34363=CARTESIAN_POINT('',(14.55,34.6639498521117,-3.98585879033799));
#34364=CARTESIAN_POINT('Origin',(-14.55,32.6768994428521,0.493790266347305));
#34365=CARTESIAN_POINT('Origin',(-22.5,34.9999999945949,6.55125051005245E-10));
#34366=CARTESIAN_POINT('Origin',(14.55,32.6156398209602,3.21167037016456));
#34367=CARTESIAN_POINT('',(14.55,32.6156398209602,3.21167037016456));
#34368=CARTESIAN_POINT('Origin',(14.55,32.6768994428521,0.493790266347305));
#34369=CARTESIAN_POINT('Origin',(-14.55,32.6768994428521,0.493790266347305));
#34370=CARTESIAN_POINT('Origin',(-14.55,37.3231005463377,-0.493790265037065));
#34371=CARTESIAN_POINT('',(-14.55,37.3843601682296,-3.21167036885432));
#34372=CARTESIAN_POINT('Origin',(14.55,37.3843601682296,-3.21167036885432));
#34373=CARTESIAN_POINT('',(14.55,37.3843601682296,-3.21167036885432));
#34374=CARTESIAN_POINT('Origin',(14.55,37.3231005463377,-0.493790265037065));
#34375=CARTESIAN_POINT('Origin',(14.55,34.6639498521117,-3.98585879033799));
#34376=CARTESIAN_POINT('Origin',(7.887499720689,31.2699373408939,2.37747721518037));
#34377=CARTESIAN_POINT('',(6.846093470689,31.0282400003182,1.24038062932732));
#34378=CARTESIAN_POINT('',(6.259999720689,31.2054847167403,2.07425145895289));
#34379=CARTESIAN_POINT('',(7.112499720689,30.9476742201263,0.861348434042974));
#34380=CARTESIAN_POINT('',(5.949999720689,31.0282400003182,1.24038062932732));
#34381=CARTESIAN_POINT('',(5.949999720689,31.0282400003182,1.24038062932732));
#34382=CARTESIAN_POINT('',(5.949999720689,30.8671084399344,0.482316238758624));
#34383=CARTESIAN_POINT('',(5.949999720689,30.8671084399344,0.482316238758624));
#34384=CARTESIAN_POINT('',(6.846093470689,30.8671084399344,0.482316238758625));
#34385=CARTESIAN_POINT('',(7.112499720689,30.8671084399344,0.482316238758625));
#34386=CARTESIAN_POINT('',(6.259999720689,30.6898637235123,-0.351554590866945));
#34387=CARTESIAN_POINT('',(6.259999720689,30.6898637235123,-0.351554590866945));
#34388=CARTESIAN_POINT('',(7.112499720689,30.8117194660525,0.221731604500634));
#34389=CARTESIAN_POINT('',(7.499999720689,30.8671084399344,0.482316238758625));
#34390=CARTESIAN_POINT('',(7.112499720689,30.6254110993588,-0.654780347094424));
#34391=CARTESIAN_POINT('',(7.112499720689,30.6254110993588,-0.654780347094424));
#34392=CARTESIAN_POINT('',(7.887499720689,30.6254110993588,-0.654780347094424));
#34393=CARTESIAN_POINT('',(7.887499720689,30.6254110993588,-0.654780347094424));
#34394=CARTESIAN_POINT('',(7.887499720689,30.8117194660525,0.221731604500634));
#34395=CARTESIAN_POINT('',(7.887499720689,30.8671084399344,0.482316238758625));
#34396=CARTESIAN_POINT('',(8.739999720689,30.6898637235123,-0.351554590866944));
#34397=CARTESIAN_POINT('',(8.739999720689,30.6898637235123,-0.351554590866944));
#34398=CARTESIAN_POINT('',(8.153905970689,30.8671084399344,0.482316238758625));
#34399=CARTESIAN_POINT('',(7.887499720689,30.9476742201263,0.861348434042974));
#34400=CARTESIAN_POINT('',(9.049999720689,30.8671084399344,0.482316238758625));
#34401=CARTESIAN_POINT('',(9.049999720689,30.8671084399344,0.482316238758625));
#34402=CARTESIAN_POINT('',(9.049999720689,31.0282400003182,1.24038062932732));
#34403=CARTESIAN_POINT('',(9.049999720689,31.0282400003182,1.24038062932732));
#34404=CARTESIAN_POINT('',(8.153905970689,31.0282400003182,1.24038062932732));
#34405=CARTESIAN_POINT('',(7.887499720689,31.0282400003182,1.24038062932732));
#34406=CARTESIAN_POINT('',(8.739999720689,31.2054847167403,2.07425145895289));
#34407=CARTESIAN_POINT('',(8.739999720689,31.2054847167403,2.07425145895289));
#34408=CARTESIAN_POINT('',(7.887499720689,31.0836289742001,1.50096526358531));
#34409=CARTESIAN_POINT('',(7.499999720689,31.0282400003182,1.24038062932732));
#34410=CARTESIAN_POINT('',(7.887499720689,31.2699373408939,2.37747721518037));
#34411=CARTESIAN_POINT('',(7.887499720689,31.2699373408939,2.37747721518037));
#34412=CARTESIAN_POINT('',(7.112499720689,31.2699373408939,2.37747721518037));
#34413=CARTESIAN_POINT('',(7.112499720689,31.2699373408939,2.37747721518037));
#34414=CARTESIAN_POINT('',(7.112499720689,31.0836289742001,1.50096526358531));
#34415=CARTESIAN_POINT('',(7.112499720689,31.0282400003182,1.24038062932732));
#34416=CARTESIAN_POINT('',(6.259999720689,31.2054847167403,2.07425145895289));
#34417=CARTESIAN_POINT('Origin',(5.949999720689,28.5195541981733,0.981304296721248));
#34418=CARTESIAN_POINT('',(5.949999720689,28.5195541981733,0.981304296721248));
#34419=CARTESIAN_POINT('',(5.949999720689,28.6806857585571,1.73936868728995));
#34420=CARTESIAN_POINT('Origin',(7.112499720689,28.5195541981733,0.981304296721249));
#34421=CARTESIAN_POINT('',(6.846093470689,28.5195541981733,0.981304296721249));
#34422=CARTESIAN_POINT('Origin',(6.259999720689,28.3423094817512,0.14743346709568));
#34423=CARTESIAN_POINT('',(6.259999720689,28.3423094817512,0.14743346709568));
#34424=CARTESIAN_POINT('Origin',(7.499999720689,28.5195541981733,0.981304296721249));
#34425=CARTESIAN_POINT('',(7.112499720689,28.4641652242914,0.720719662463258));
#34426=CARTESIAN_POINT('Origin',(7.112499720689,28.2778568575977,-0.1557922891318));
#34427=CARTESIAN_POINT('',(7.112499720689,28.2778568575977,-0.1557922891318));
#34428=CARTESIAN_POINT('Origin',(7.887499720689,28.2778568575977,-0.1557922891318));
#34429=CARTESIAN_POINT('',(7.887499720689,28.2778568575977,-0.1557922891318));
#34430=CARTESIAN_POINT('Origin',(7.887499720689,28.5195541981733,0.981304296721249));
#34431=CARTESIAN_POINT('',(7.887499720689,28.4641652242914,0.720719662463259));
#34432=CARTESIAN_POINT('Origin',(8.739999720689,28.3423094817512,0.14743346709568));
#34433=CARTESIAN_POINT('',(8.739999720689,28.3423094817512,0.14743346709568));
#34434=CARTESIAN_POINT('Origin',(7.887499720689,28.6001199783652,1.3603364920056));
#34435=CARTESIAN_POINT('',(8.153905970689,28.5195541981733,0.981304296721249));
#34436=CARTESIAN_POINT('Origin',(9.049999720689,28.5195541981733,0.981304296721249));
#34437=CARTESIAN_POINT('',(9.049999720689,28.5195541981733,0.981304296721249));
#34438=CARTESIAN_POINT('Origin',(9.049999720689,28.6806857585571,1.73936868728995));
#34439=CARTESIAN_POINT('',(9.049999720689,28.6806857585571,1.73936868728995));
#34440=CARTESIAN_POINT('Origin',(7.887499720689,28.6806857585571,1.73936868728995));
#34441=CARTESIAN_POINT('',(8.153905970689,28.6806857585571,1.73936868728995));
#34442=CARTESIAN_POINT('Origin',(8.739999720689,28.8579304749792,2.57323951691552));
#34443=CARTESIAN_POINT('',(8.739999720689,28.8579304749792,2.57323951691552));
#34444=CARTESIAN_POINT('Origin',(7.499999720689,28.6806857585571,1.73936868728995));
#34445=CARTESIAN_POINT('',(7.887499720689,28.736074732439,1.99995332154794));
#34446=CARTESIAN_POINT('Origin',(7.887499720689,28.9223830991327,2.876465273143));
#34447=CARTESIAN_POINT('',(7.887499720689,28.9223830991327,2.876465273143));
#34448=CARTESIAN_POINT('Origin',(7.112499720689,28.9223830991327,2.876465273143));
#34449=CARTESIAN_POINT('',(7.112499720689,28.9223830991327,2.876465273143));
#34450=CARTESIAN_POINT('Origin',(7.112499720689,28.6806857585571,1.73936868728995));
#34451=CARTESIAN_POINT('',(7.112499720689,28.736074732439,1.99995332154794));
#34452=CARTESIAN_POINT('Origin',(6.259999720689,28.8579304749792,2.57323951691552));
#34453=CARTESIAN_POINT('',(6.259999720689,28.8579304749792,2.57323951691552));
#34454=CARTESIAN_POINT('Origin',(7.112499720689,28.6001199783652,1.3603364920056));
#34455=CARTESIAN_POINT('',(6.846093470689,28.6806857585571,1.73936868728995));
#34456=CARTESIAN_POINT('Origin',(5.949999720689,28.6806857585571,1.73936868728995));
#34457=CARTESIAN_POINT('Origin',(4.499999720689,32.0655571923935,0.6237350731084));
#34458=CARTESIAN_POINT('Origin',(4.499999720689,32.0655571923935,0.6237350731084));
#34459=CARTESIAN_POINT('Origin',(0.,34.510926194228,0.103955846064));
#34460=CARTESIAN_POINT('Origin',(5.19584375524573E-13,34.5109261942278,
0.103955846063327));
#34461=CARTESIAN_POINT('Origin',(0.,35.4890737949618,-0.10395584475376));
#34462=CARTESIAN_POINT('Origin',(2.55351295663786E-13,35.4890737949617,
-0.103955844754159));
#34463=CARTESIAN_POINT('Origin',(0.,34.510926194228,0.103955846064));
#34464=CARTESIAN_POINT('Origin',(1.32155929348462E-13,34.5109261942281,
0.103955846064179));
#34465=CARTESIAN_POINT('Ctrl Pts',(0.,32.3703984326954,-14.7761698557608));
#34466=CARTESIAN_POINT('Ctrl Pts',(0.,31.1966213118148,-14.5266758267795));
#34467=CARTESIAN_POINT('Ctrl Pts',(-29.,32.3703984326954,-14.7761698557608));
#34468=CARTESIAN_POINT('Ctrl Pts',(-29.,31.1966213118148,-14.5266758267795));
#34469=CARTESIAN_POINT('Ctrl Pts',(-29.,38.6077491572282,14.5682581662533));
#34470=CARTESIAN_POINT('Ctrl Pts',(-29.,37.4339720363476,14.8177521952346));
#34471=CARTESIAN_POINT('Ctrl Pts',(-1.77573785876366E-15,38.6077491572282,
14.5682581662533));
#34472=CARTESIAN_POINT('Ctrl Pts',(-1.77573785876366E-15,37.4339720363476,
14.8177521952346));
#34473=CARTESIAN_POINT('Origin',(1.88970922978163E-13,35.4890737949618,
-0.103955844753516));
#34474=CARTESIAN_POINT('Origin',(0.,35.4890737949618,-0.10395584475376));
#62950=UNCERTAINTY_MEASURE_WITH_UNIT(LENGTH_MEASURE(0.01),#62975,
'DISTANCE_ACCURACY_VALUE',
'Maximum model space distance between geometric entities at asserted c
onnectivities');
#62960=UNCERTAINTY_MEASURE_WITH_UNIT(LENGTH_MEASURE(0.01),#62975,
'DISTANCE_ACCURACY_VALUE',
'Maximum model space distance between geometric entities at asserted c
onnectivities');
#62964=(
GEOMETRIC_REPRESENTATION_CONTEXT(3)
GLOBAL_UNCERTAINTY_ASSIGNED_CONTEXT((#62950))
GLOBAL_UNIT_ASSIGNED_CONTEXT((#62975,#62977,#62978))
REPRESENTATION_CONTEXT('','3D')
);
#62974=(
GEOMETRIC_REPRESENTATION_CONTEXT(3)
GLOBAL_UNCERTAINTY_ASSIGNED_CONTEXT((#62960))
GLOBAL_UNIT_ASSIGNED_CONTEXT((#62975,#62977,#62978))
REPRESENTATION_CONTEXT('','3D')
);
#62975=(
LENGTH_UNIT()
NAMED_UNIT(*)
SI_UNIT(.MILLI.,.METRE.)
);
#62977=(
NAMED_UNIT(*)
PLANE_ANGLE_UNIT()
SI_UNIT($,.RADIAN.)
);
#62978=(
NAMED_UNIT(*)
SI_UNIT($,.STERADIAN.)
SOLID_ANGLE_UNIT()
);
#62982=SHAPE_DEFINITION_REPRESENTATION(#62995,#63023);
#62995=PRODUCT_DEFINITION_SHAPE('',$,#63037);
#63023=SHAPE_REPRESENTATION('',(#15531),#62964);
#63033=PRODUCT_DEFINITION_CONTEXT('part definition',#63074,'design');
#63037=PRODUCT_DEFINITION('Throttle Shaft & Butterfly Valve',
'Throttle Shaft & Butterfly Valve',#63050,#63033);
#63050=PRODUCT_DEFINITION_FORMATION('',$,#63079);
#63074=APPLICATION_CONTEXT(
'Core Data for Automotive Mechanical Design Process');
#63075=PRODUCT_CONTEXT('part definition',#63074,'mechanical');
#63079=PRODUCT('Throttle Shaft & Butterfly Valve',
'Throttle Shaft & Butterfly Valve',$,(#63075));
#63090=PRESENTATION_STYLE_ASSIGNMENT((#63092));
#63092=SURFACE_STYLE_USAGE(.BOTH.,#63094);
#63094=SURFACE_SIDE_STYLE('',(#63096));
#63096=SURFACE_STYLE_FILL_AREA(#63098);
#63098=FILL_AREA_STYLE('Opaque(202,209,238)',(#63100));
#63100=FILL_AREA_STYLE_COLOUR('Opaque(202,209,238)',#63102);
#63102=COLOUR_RGB('Opaque(202,209,238)', 0.66274510, 0.83137255, 0.94901961);
ENDSEC;
END-ISO-10303-21;
